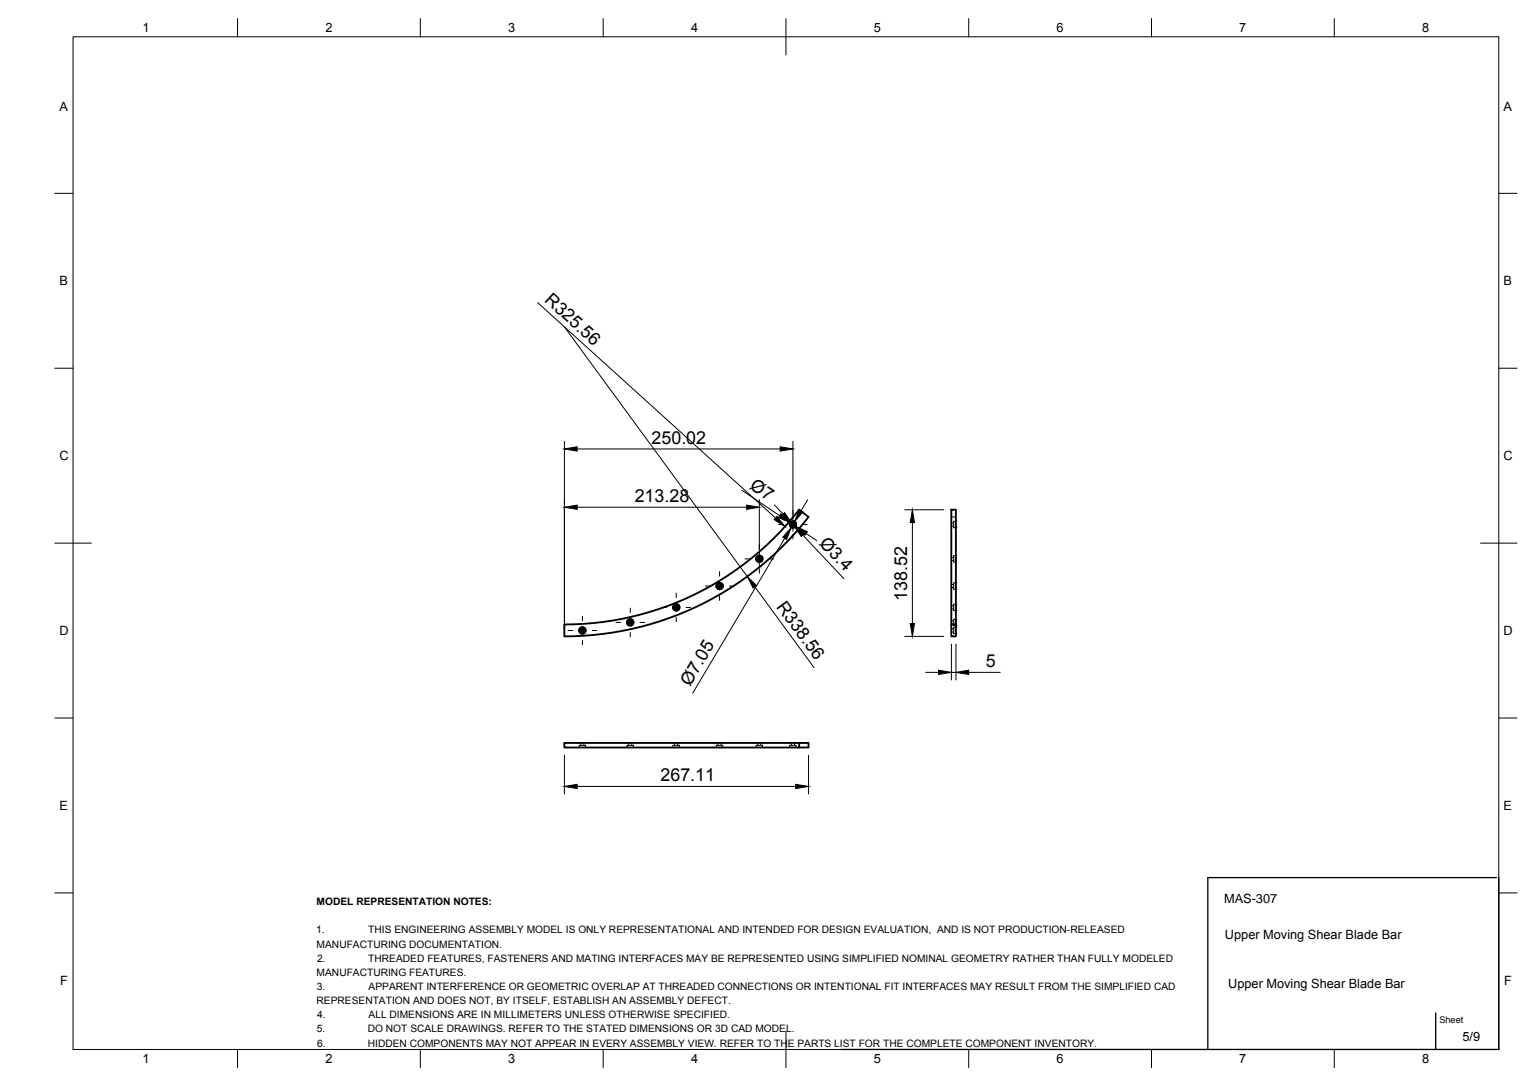
ISO-10303-21;
HEADER;
FILE_DESCRIPTION (('STEP AP214'),
    '1' );
FILE_NAME ('Upper Moving Shear Blade Bar.step',
    '2026-10-06T07:34:29',
    ( '' ),
    ( '' ),
    'SwSTEP 2.0',
    'SolidWorks 2025',
    '' );
FILE_SCHEMA (( 'AUTOMOTIVE_DESIGN' ));
ENDSEC;

DATA;
#5=CIRCLE ( 'NONE', #1538, 3.525000000000000355 ) ;
#15=CARTESIAN_POINT ( 'NONE',  ( 66.76535645333922275, 38.79159067395544014, 7.600000000000002309 ) ) ;
#20=DIRECTION ( 'NONE',  ( -0.000000000000000000, -0.000000000000000000, 1.000000000000000000 ) ) ;
#38=DIRECTION ( 'NONE',  ( 1.000000000000000000, 0.000000000000000000, 0.000000000000000000 ) ) ;
#47=CARTESIAN_POINT ( 'NONE',  ( 70.26535645333922275, 38.79159067395544014, 10.00000000000000178 ) ) ;
#51=DIRECTION ( 'NONE',  ( 1.000000000000000000, 0.000000000000000000, 0.000000000000000000 ) ) ;
#52=CARTESIAN_POINT ( 'NONE',  ( -36.49899788034579018, 48.72489408690345414, 5.000000000000000000 ) ) ;
#60=EDGE_CURVE ( 'NONE', #13786, #6568, #5831, .T. ) ;
#63=ORIENTED_EDGE ( 'NONE', *, *, #11844, .T. ) ;
#76=CARTESIAN_POINT ( 'NONE',  ( 70.26535645333922275, 38.79159067395544014, 7.600000000000002309 ) ) ;
#82=DIRECTION ( 'NONE',  ( -0.000000000000000000, -0.000000000000000000, 1.000000000000000000 ) ) ;
#84=DIRECTION ( 'NONE',  ( 1.000000000000000000, 0.000000000000000000, 0.000000000000000000 ) ) ;
#90=LINE ( 'NONE', #10937, #11841 ) ;
#97=CARTESIAN_POINT ( 'NONE',  ( -34.79899788034579444, 48.72489408690345414, 10.00000000000000178 ) ) ;
#109=DIRECTION ( 'NONE',  ( -0.000000000000000000, -0.000000000000000000, 1.000000000000000000 ) ) ;
#120=ADVANCED_FACE ( 'NONE', ( #7198 ), #13161, .F. ) ;
#143=ORIENTED_EDGE ( 'NONE', *, *, #13656, .T. ) ;
#158=VERTEX_POINT ( 'NONE', #7269 ) ;
#175=ORIENTED_EDGE ( 'NONE', *, *, #1719, .F. ) ;
#184=DIRECTION ( 'NONE',  ( -0.000000000000000000, -0.000000000000000000, 1.000000000000000000 ) ) ;
#191=AXIS2_PLACEMENT_3D ( 'NONE', #8581, #13373, #8730 ) ;
#197=DIRECTION ( 'NONE',  ( 1.000000000000000000, 0.000000000000000000, 0.000000000000000000 ) ) ;
#204=DIRECTION ( 'NONE',  ( 1.000000000000000000, 0.000000000000000000, 0.000000000000000000 ) ) ;
#218=EDGE_CURVE ( 'NONE', #11968, #7924, #4346, .T. ) ;
#256=VERTEX_POINT ( 'NONE', #7495 ) ;
#266=DIRECTION ( 'NONE',  ( -0.000000000000000000, -0.000000000000000000, 1.000000000000000000 ) ) ;
#269=MANIFOLD_SOLID_BREP ( 'Move Face1', #9158 ) ;
#270=LINE ( 'NONE', #1701, #14484 ) ;
#273=VECTOR ( 'NONE', #10509, 1000.000000000000000 ) ;
#287=FACE_OUTER_BOUND ( 'NONE', #14918, .T. ) ;
#302=DIRECTION ( 'NONE',  ( 1.000000000000000000, 0.000000000000000000, 0.000000000000000000 ) ) ;
#342=FACE_OUTER_BOUND ( 'NONE', #1259, .T. ) ;
#352=EDGE_LOOP ( 'NONE', ( #9480, #1820, #544, #3677 ) ) ;
#354=DIRECTION ( 'NONE',  ( -0.000000000000000000, -0.000000000000000000, 1.000000000000000000 ) ) ;
#372=FACE_OUTER_BOUND ( 'NONE', #12651, .T. ) ;
#376=CARTESIAN_POINT ( 'NONE',  ( 19.11029453487719110, 40.04259805664093363, 7.600000000000002309 ) ) ;
#388=FACE_BOUND ( 'NONE', #1673, .T. ) ;
#407=DIRECTION ( 'NONE',  ( -0.000000000000000000, -0.000000000000000000, 1.000000000000000000 ) ) ;
#412=DIRECTION ( 'NONE',  ( 1.000000000000000000, 0.000000000000000000, 0.000000000000000000 ) ) ;
#414=FACE_OUTER_BOUND ( 'NONE', #14323, .T. ) ;
#418=ADVANCED_FACE ( 'NONE', ( #10869 ), #4776, .F. ) ;
#430=FACE_OUTER_BOUND ( 'NONE', #4920, .T. ) ;
#439=ADVANCED_FACE ( 'NONE', ( #5527 ), #13887, .F. ) ;
#440=DIRECTION ( 'NONE',  ( 1.000000000000000000, 0.000000000000000000, 0.000000000000000000 ) ) ;
#447=ORIENTED_EDGE ( 'NONE', *, *, #8449, .T. ) ;
#452=CARTESIAN_POINT ( 'NONE',  ( 122.5806775638430253, 45.00321902537314145, 7.600000000000002309 ) ) ;
#453=AXIS2_PLACEMENT_3D ( 'NONE', #12309, #7594, #7753 ) ;
#454=VECTOR ( 'NONE', #11405, 1000.000000000000114 ) ;
#457=VERTEX_POINT ( 'NONE', #4861 ) ;
#475=DIRECTION ( 'NONE',  ( -1.000000000000000000, 0.000000000000000000, 0.000000000000000000 ) ) ;
#492=DIRECTION ( 'NONE',  ( 1.000000000000000000, 0.000000000000000000, 0.000000000000000000 ) ) ;
#493=CARTESIAN_POINT ( 'NONE',  ( -33.09899788034579160, 48.72489408690345414, 7.600000000000002309 ) ) ;
#507=LINE ( 'NONE', #14731, #10105 ) ;
#508=ORIENTED_EDGE ( 'NONE', *, *, #8880, .F. ) ;
#509=EDGE_LOOP ( 'NONE', ( #9428, #2544 ) ) ;
#511=CARTESIAN_POINT ( 'NONE',  ( 124.2806775638430281, 45.00321902537314145, 5.000000000000000000 ) ) ;
#538=CARTESIAN_POINT ( 'NONE',  ( 70.26535645333922275, 38.79159067395544014, 10.00000000000000178 ) ) ;
#540=FACE_OUTER_BOUND ( 'NONE', #6429, .T. ) ;
#544=ORIENTED_EDGE ( 'NONE', *, *, #8820, .T. ) ;
#551=ORIENTED_EDGE ( 'NONE', *, *, #13799, .F. ) ;
#556=SHAPE_REPRESENTATION ( 'Upper Moving Shear Blade Bar', ( #12337 ), #11555 ) ;
#569=DIRECTION ( 'NONE',  ( 1.000000000000000000, 0.000000000000000000, 0.000000000000000000 ) ) ;
#574=UNCERTAINTY_MEASURE_WITH_UNIT (LENGTH_MEASURE( 1.000000000000000082E-05 ), #14890, 'distance_accuracy_value', 'NONE');
#589=ORIENTED_EDGE ( 'NONE', *, *, #6377, .F. ) ;
#601=CIRCLE ( 'NONE', #13716, 3.500000000000003109 ) ;
#606=AXIS2_PLACEMENT_3D ( 'NONE', #2740, #184, #1548 ) ;
#622=EDGE_CURVE ( 'NONE', #2293, #7132, #13393, .T. ) ;
#633=CARTESIAN_POINT ( 'NONE',  ( -31.27399788034579586, 48.72489408690345414, 10.00000000000000178 ) ) ;
#656=CARTESIAN_POINT ( 'NONE',  ( -33.09899788034579871, 48.72489408690345414, 10.00000000000000178 ) ) ;
#675=DIRECTION ( 'NONE',  ( -0.000000000000000000, -0.000000000000000000, 1.000000000000000000 ) ) ;
#705=EDGE_CURVE ( 'NONE', #14207, #5229, #14437, .T. ) ;
#734=EDGE_CURVE ( 'NONE', #12823, #5329, #1812, .T. ) ;
#738=CARTESIAN_POINT ( 'NONE',  ( -105.7032403413611661, 68.63699971342407480, 10.00000000000000178 ) ) ;
#748=EDGE_LOOP ( 'NONE', ( #9743, #1718 ) ) ;
#749=ORIENTED_EDGE ( 'NONE', *, *, #705, .F. ) ;
#752=LINE ( 'NONE', #5511, #3482 ) ;
#753=CIRCLE ( 'NONE', #1005, 3.525000000000000355 ) ;
#754=AXIS2_PLACEMENT_3D ( 'NONE', #3682, #1381, #6219 ) ;
#762=AXIS2_PLACEMENT_3D ( 'NONE', #942, #1027, #8085 ) ;
#771=CARTESIAN_POINT ( 'NONE',  ( -85.27455057502459113, 65.19100426474074084, 10.00000000000000178 ) ) ;
#772=ORIENTED_EDGE ( 'NONE', *, *, #9707, .F. ) ;
#795=LINE ( 'NONE', #4513, #5561 ) ;
#803=DIRECTION ( 'NONE',  ( -0.000000000000000000, -0.000000000000000000, 1.000000000000000000 ) ) ;
#810=VERTEX_POINT ( 'NONE', #13328 ) ;
#828=VERTEX_POINT ( 'NONE', #6562 ) ;
#834=DIRECTION ( 'NONE',  ( -0.000000000000000000, 0.000000000000000000, 1.000000000000000000 ) ) ;
#837=VECTOR ( 'NONE', #9700, 1000.000000000000000 ) ;
#845=DIRECTION ( 'NONE',  ( 1.000000000000000000, 0.000000000000000000, 0.000000000000000000 ) ) ;
#847=AXIS2_PLACEMENT_3D ( 'NONE', #10566, #8058, #12846 ) ;
#872=CIRCLE ( 'NONE', #11474, 3.500000000000003109 ) ;
#875=DIRECTION ( 'NONE',  ( 1.000000000000000000, 0.000000000000000000, 0.000000000000000000 ) ) ;
#880=ORIENTED_EDGE ( 'NONE', *, *, #9050, .T. ) ;
#883=CARTESIAN_POINT ( 'NONE',  ( -31.27399788034579586, 48.72489408690345414, 10.00000000000000178 ) ) ;
#900=DIRECTION ( 'NONE',  ( -0.000000000000000000, -0.000000000000000000, -1.000000000000000000 ) ) ;
#911=ADVANCED_FACE ( 'NONE', ( #11682 ), #8886, .F. ) ;
#933=DIRECTION ( 'NONE',  ( -0.000000000000000000, -0.000000000000000000, 1.000000000000000000 ) ) ;
#935=VERTEX_POINT ( 'NONE', #2196 ) ;
#938=EDGE_CURVE ( 'NONE', #2958, #9645, #5088, .T. ) ;
#940=ORIENTED_EDGE ( 'NONE', *, *, #1886, .F. ) ;
#942=CARTESIAN_POINT ( 'NONE',  ( 172.5293059057019889, 61.25683321636181233, 7.600000000000002309 ) ) ;
#956=VERTEX_POINT ( 'NONE', #3310 ) ;
#976=EDGE_LOOP ( 'NONE', ( #1480, #10214, #12873, #13520 ) ) ;
#977=CARTESIAN_POINT ( 'NONE',  ( 71.96535645333923981, 38.79159067395544014, 7.600000000000002309 ) ) ;
#997=CARTESIAN_POINT ( 'NONE',  ( 176.0293059057019889, 61.25683321636181233, 7.600000000000002309 ) ) ;
#1005=AXIS2_PLACEMENT_3D ( 'NONE', #12927, #3078, #15361 ) ;
#1027=DIRECTION ( 'NONE',  ( -0.000000000000000000, -0.000000000000000000, 1.000000000000000000 ) ) ;
#1029=DIRECTION ( 'NONE',  ( 1.000000000000000000, 0.000000000000000000, 0.000000000000000000 ) ) ;
#1085=CARTESIAN_POINT ( 'NONE',  ( -34.79899788034579444, 48.72489408690345414, 7.600000000000002309 ) ) ;
#1096=EDGE_LOOP ( 'NONE', ( #7071, #14748 ) ) ;
#1098=VERTEX_POINT ( 'NONE', #10967 ) ;
#1117=ORIENTED_EDGE ( 'NONE', *, *, #218, .F. ) ;
#1118=LINE ( 'NONE', #14294, #8578 ) ;
#1125=EDGE_LOOP ( 'NONE', ( #7007, #5807 ) ) ;
#1139=FACE_OUTER_BOUND ( 'NONE', #12303, .T. ) ;
#1162=ORIENTED_EDGE ( 'NONE', *, *, #10778, .F. ) ;
#1167=FACE_BOUND ( 'NONE', #3663, .T. ) ;
#1168=CARTESIAN_POINT ( 'NONE',  ( 51.07686401294030532, 368.7106150007013525, 10.00000000000000178 ) ) ;
#1171=ORIENTED_EDGE ( 'NONE', *, *, #5302, .T. ) ;
#1179=CARTESIAN_POINT ( 'NONE',  ( -34.79899788034579444, 48.72489408690345414, 5.000000000000000000 ) ) ;
#1180=CARTESIAN_POINT ( 'NONE',  ( 119.0806775638430253, 45.00321902537314145, 10.00000000000000178 ) ) ;
#1185=DIRECTION ( 'NONE',  ( -0.000000000000000000, -0.000000000000000000, 1.000000000000000000 ) ) ;
#1189=CIRCLE ( 'NONE', #6262, 3.500000000000003109 ) ;
#1196=CIRCLE ( 'NONE', #10531, 1.700000000000007061 ) ;
#1204=ORIENTED_EDGE ( 'NONE', *, *, #5302, .F. ) ;
#1211=DIRECTION ( 'NONE',  ( -1.000000000000000000, 0.000000000000000000, 0.000000000000000000 ) ) ;
#1218=AXIS2_PLACEMENT_3D ( 'NONE', #1179, #3479, #13179 ) ;
#1222=ORIENTED_EDGE ( 'NONE', *, *, #4363, .T. ) ;
#1226=DIRECTION ( 'NONE',  ( -0.000000000000000000, -0.000000000000000000, 1.000000000000000000 ) ) ;
#1227=FACE_OUTER_BOUND ( 'NONE', #14901, .T. ) ;
#1256=CARTESIAN_POINT ( 'NONE',  ( 170.8293059057019718, 61.25683321636181233, 10.00000000000000178 ) ) ;
#1259=EDGE_LOOP ( 'NONE', ( #5459, #10454, #4600, #3411 ) ) ;
#1274=EDGE_LOOP ( 'NONE', ( #3424, #1499, #2007, #2831 ) ) ;
#1275=CARTESIAN_POINT ( 'NONE',  ( 17.41029453487719181, 40.04259805664093363, 7.600000000000002309 ) ) ;
#1286=CARTESIAN_POINT ( 'NONE',  ( 124.2806775638430281, 45.00321902537314145, 7.600000000000002309 ) ) ;
#1294=CARTESIAN_POINT ( 'NONE',  ( -81.74955057502458544, 65.19100426474074084, 10.00000000000000178 ) ) ;
#1305=DIRECTION ( 'NONE',  ( 1.000000000000000000, 0.000000000000000000, 0.000000000000000000 ) ) ;
#1325=FACE_BOUND ( 'NONE', #9221, .T. ) ;
#1341=CARTESIAN_POINT ( 'NONE',  ( 70.26535645333922275, 38.79159067395544014, 10.00000000000000178 ) ) ;
#1349=DIRECTION ( 'NONE',  ( -0.000000000000000000, -0.000000000000000000, -1.000000000000000000 ) ) ;
#1381=DIRECTION ( 'NONE',  ( -0.000000000000000000, -0.000000000000000000, 1.000000000000000000 ) ) ;
#1383=DIRECTION ( 'NONE',  ( 1.000000000000000000, 0.000000000000000000, 0.000000000000000000 ) ) ;
#1393=CARTESIAN_POINT ( 'NONE',  ( -31.29899788034579089, 48.72489408690345414, 7.600000000000002309 ) ) ;
#1396=CARTESIAN_POINT ( 'NONE',  ( 70.26535645333922275, 38.79159067395544014, 5.000000000000000000 ) ) ;
#1420=CARTESIAN_POINT ( 'NONE',  ( -34.79899788034579444, 48.72489408690345414, 10.00000000000000178 ) ) ;
#1426=VERTEX_POINT ( 'NONE', #8206 ) ;
#1446=DIRECTION ( 'NONE',  ( 1.000000000000000000, 0.000000000000000000, 0.000000000000000000 ) ) ;
#1463=ORIENTED_EDGE ( 'NONE', *, *, #6997, .F. ) ;
#1472=CARTESIAN_POINT ( 'NONE',  ( 122.5806775638430253, 45.00321902537314145, 10.00000000000000178 ) ) ;
#1476=CARTESIAN_POINT ( 'NONE',  ( -86.97455057502459397, 65.19100426474074084, 10.00000000000000178 ) ) ;
#1480=ORIENTED_EDGE ( 'NONE', *, *, #734, .F. ) ;
#1494=ORIENTED_EDGE ( 'NONE', *, *, #10730, .T. ) ;
#1499=ORIENTED_EDGE ( 'NONE', *, *, #9175, .T. ) ;
#1507=LINE ( 'NONE', #10999, #2120 ) ;
#1511=LINE ( 'NONE', #11231, #6713 ) ;
#1538=AXIS2_PLACEMENT_3D ( 'NONE', #14552, #13293, #7325 ) ;
#1548=DIRECTION ( 'NONE',  ( 1.000000000000000000, 0.000000000000000000, 0.000000000000000000 ) ) ;
#1553=ORIENTED_EDGE ( 'NONE', *, *, #12044, .T. ) ;
#1554=LINE ( 'NONE', #1787, #12369 ) ;
#1604=EDGE_CURVE ( 'NONE', #956, #13999, #11477, .T. ) ;
#1613=AXIS2_PLACEMENT_3D ( 'NONE', #12528, #5520, #1722 ) ;
#1620=ORIENTED_EDGE ( 'NONE', *, *, #11583, .F. ) ;
#1633=EDGE_CURVE ( 'NONE', #8949, #7872, #9856, .T. ) ;
#1634=AXIS2_PLACEMENT_3D ( 'NONE', #15188, #12908, #6927 ) ;
#1641=DIRECTION ( 'NONE',  ( -0.000000000000000000, 0.000000000000000000, 1.000000000000000000 ) ) ;
#1645=CYLINDRICAL_SURFACE ( 'NONE', #5383, 3.499999999999999556 ) ;
#1660=FACE_OUTER_BOUND ( 'NONE', #8338, .T. ) ;
#1673=EDGE_LOOP ( 'NONE', ( #11669, #7615 ) ) ;
#1682=EDGE_CURVE ( 'NONE', #5329, #12823, #13351, .T. ) ;
#1697=DIRECTION ( 'NONE',  ( -0.000000000000000000, -0.000000000000000000, 1.000000000000000000 ) ) ;
#1698=CIRCLE ( 'NONE', #3471, 3.499999999999999556 ) ;
#1701=CARTESIAN_POINT ( 'NONE',  ( -31.29899788034579089, 48.72489408690345414, 10.00000000000000178 ) ) ;
#1706=PRODUCT_DEFINITION_SHAPE ( 'NONE', 'NONE',  #4976 ) ;
#1713=AXIS2_PLACEMENT_3D ( 'NONE', #5111, #12137, #8746 ) ;
#1718=ORIENTED_EDGE ( 'NONE', *, *, #4489, .F. ) ;
#1719=EDGE_CURVE ( 'NONE', #3938, #7406, #5234, .T. ) ;
#1722=DIRECTION ( 'NONE',  ( 1.000000000000000000, 0.000000000000000000, 0.000000000000000000 ) ) ;
#1726=EDGE_LOOP ( 'NONE', ( #15460, #12803, #6817, #4219 ) ) ;
#1741=VECTOR ( 'NONE', #7234, 1000.000000000000000 ) ;
#1759=DIRECTION ( 'NONE',  ( 1.000000000000000000, 0.000000000000000000, 0.000000000000000000 ) ) ;
#1781=CARTESIAN_POINT ( 'NONE',  ( 172.5293059057019889, 61.25683321636181233, 10.00000000000000178 ) ) ;
#1783=CARTESIAN_POINT ( 'NONE',  ( 13.91029453487719181, 40.04259805664093363, 7.600000000000002309 ) ) ;
#1787=CARTESIAN_POINT ( 'NONE',  ( 66.76535645333922275, 38.79159067395544014, 10.00000000000000178 ) ) ;
#1812=CIRCLE ( 'NONE', #6623, 3.499999999999996003 ) ;
#1816=AXIS2_PLACEMENT_3D ( 'NONE', #3969, #8888, #13595 ) ;
#1820=ORIENTED_EDGE ( 'NONE', *, *, #9243, .T. ) ;
#1822=MECHANICAL_DESIGN_GEOMETRIC_PRESENTATION_REPRESENTATION('',(#4599),#12887);
#1834=DIRECTION ( 'NONE',  ( 0.000000000000000000, 0.000000000000000000, -1.000000000000000000 ) ) ;
#1842=ORIENTED_EDGE ( 'NONE', *, *, #14993, .F. ) ;
#1859=EDGE_LOOP ( 'NONE', ( #2042, #2199, #11914, #1842 ) ) ;
#1861=EDGE_CURVE ( 'NONE', #12197, #8972, #3037, .T. ) ;
#1862=ORIENTED_EDGE ( 'NONE', *, *, #6839, .F. ) ;
#1873=CARTESIAN_POINT ( 'NONE',  ( 174.2293059057019775, 61.25683321636181233, 5.000000000000000000 ) ) ;
#1886=EDGE_CURVE ( 'NONE', #8972, #935, #795, .T. ) ;
#1903=CARTESIAN_POINT ( 'NONE',  ( 172.5293059057019889, 61.25683321636181233, 7.600000000000002309 ) ) ;
#1937=ORIENTED_EDGE ( 'NONE', *, *, #4142, .F. ) ;
#1947=EDGE_CURVE ( 'NONE', #11858, #256, #2789, .T. ) ;
#1974=AXIS2_PLACEMENT_3D ( 'NONE', #14287, #2218, #11936 ) ;
#1978=LINE ( 'NONE', #633, #12056 ) ;
#1981=ORIENTED_EDGE ( 'NONE', *, *, #8820, .F. ) ;
#1987=ADVANCED_FACE ( 'NONE', ( #6101 ), #7291, .F. ) ;
#2001=EDGE_LOOP ( 'NONE', ( #3858, #3321, #12575, #4549 ) ) ;
#2002=AXIS2_PLACEMENT_3D ( 'NONE', #2956, #8720, #7775 ) ;
#2007=ORIENTED_EDGE ( 'NONE', *, *, #2102, .T. ) ;
#2039=EDGE_CURVE ( 'NONE', #7454, #8789, #10609, .T. ) ;
#2042=ORIENTED_EDGE ( 'NONE', *, *, #1947, .F. ) ;
#2059=AXIS2_PLACEMENT_3D ( 'NONE', #15441, #9540, #845 ) ;
#2074=ORIENTED_EDGE ( 'NONE', *, *, #6696, .F. ) ;
#2085=AXIS2_PLACEMENT_3D ( 'NONE', #10680, #1185, #12089 ) ;
#2096=DIRECTION ( 'NONE',  ( 1.000000000000000000, 0.000000000000000000, 0.000000000000000000 ) ) ;
#2102=EDGE_CURVE ( 'NONE', #3731, #7373, #13620, .T. ) ;
#2120=VECTOR ( 'NONE', #1349, 1000.000000000000000 ) ;
#2126=CARTESIAN_POINT ( 'NONE',  ( 70.26535645333922275, 38.79159067395544014, 7.600000000000002309 ) ) ;
#2141=CIRCLE ( 'NONE', #3913, 1.700000000000000178 ) ;
#2148=ADVANCED_FACE ( 'NONE', ( #12468 ), #14629, .F. ) ;
#2150=VERTEX_POINT ( 'NONE', #376 ) ;
#2172=PLANE ( 'NONE',  #4664 ) ;
#2175=LINE ( 'NONE', #4545, #12545 ) ;
#2181=ORIENTED_EDGE ( 'NONE', *, *, #60, .F. ) ;
#2184=CARTESIAN_POINT ( 'NONE',  ( 0.000000000000000000, 0.000000000000000000, 10.00000000000000178 ) ) ;
#2189=EDGE_CURVE ( 'NONE', #12185, #15218, #2286, .T. ) ;
#2195=CARTESIAN_POINT ( 'NONE',  ( 124.2806775638430281, 45.00321902537314145, 10.00000000000000178 ) ) ;
#2196=CARTESIAN_POINT ( 'NONE',  ( -81.77455057502459113, 65.19100426474074084, 9.975000000000001421 ) ) ;
#2199=ORIENTED_EDGE ( 'NONE', *, *, #12619, .T. ) ;
#2201=CIRCLE ( 'NONE', #13024, 1.700000000000007061 ) ;
#2218=DIRECTION ( 'NONE',  ( -0.000000000000000000, -0.000000000000000000, 1.000000000000000000 ) ) ;
#2237=ORIENTED_EDGE ( 'NONE', *, *, #11806, .T. ) ;
#2249=EDGE_LOOP ( 'NONE', ( #9218, #10170, #8571, #13907 ) ) ;
#2257=AXIS2_PLACEMENT_3D ( 'NONE', #12770, #9315, #9238 ) ;
#2279=CARTESIAN_POINT ( 'NONE',  ( 186.1005832062958234, 72.46888774096882457, 10.00000000000000178 ) ) ;
#2286=CIRCLE ( 'NONE', #9349, 3.500000000000003109 ) ;
#2293=VERTEX_POINT ( 'NONE', #3231 ) ;
#2307=VECTOR ( 'NONE', #6012, 1000.000000000000000 ) ;
#2311=FACE_BOUND ( 'NONE', #3877, .T. ) ;
#2335=CARTESIAN_POINT ( 'NONE',  ( 13.91029453487719181, 40.04259805664093363, 9.975000000000001421 ) ) ;
#2342=EDGE_LOOP ( 'NONE', ( #3842, #7278 ) ) ;
#2387=EDGE_CURVE ( 'NONE', #7406, #810, #9610, .T. ) ;
#2391=VECTOR ( 'NONE', #14651, 1000.000000000000000 ) ;
#2432=ORIENTED_EDGE ( 'NONE', *, *, #13357, .T. ) ;
#2433=EDGE_CURVE ( 'NONE', #10355, #6706, #5971, .T. ) ;
#2437=CYLINDRICAL_SURFACE ( 'NONE', #10901, 3.500000000000003109 ) ;
#2451=ORIENTED_EDGE ( 'NONE', *, *, #7116, .T. ) ;
#2487=FACE_BOUND ( 'NONE', #4495, .T. ) ;
#2495=CIRCLE ( 'NONE', #3505, 3.500000000000003109 ) ;
#2497=DIRECTION ( 'NONE',  ( -0.000000000000000000, -0.000000000000000000, 1.000000000000000000 ) ) ;
#2506=CARTESIAN_POINT ( 'NONE',  ( 13.91029453487719181, 40.04259805664093363, 10.00000000000000178 ) ) ;
#2512=ADVANCED_FACE ( 'NONE', ( #13319, #1167, #1325, #5997, #3781, #4967, #10818 ), #15607, .F. ) ;
#2519=CIRCLE ( 'NONE', #9844, 1.700000000000000178 ) ;
#2524=ORIENTED_EDGE ( 'NONE', *, *, #1604, .F. ) ;
#2544=ORIENTED_EDGE ( 'NONE', *, *, #3841, .T. ) ;
#2558=CARTESIAN_POINT ( 'NONE',  ( -36.49899788034579728, 48.72489408690345414, 7.600000000000002309 ) ) ;
#2561=DIRECTION ( 'NONE',  ( -0.000000000000000000, -0.000000000000000000, 1.000000000000000000 ) ) ;
#2562=CARTESIAN_POINT ( 'NONE',  ( 17.41029453487719181, 40.04259805664093363, 10.00000000000000178 ) ) ;
#2619=DIRECTION ( 'NONE',  ( -0.000000000000000000, -0.000000000000000000, 1.000000000000000000 ) ) ;
#2658=DIRECTION ( 'NONE',  ( 1.000000000000000000, 0.000000000000000000, 0.000000000000000000 ) ) ;
#2659=DIRECTION ( 'NONE',  ( 1.000000000000000000, 0.000000000000000000, 0.000000000000000000 ) ) ;
#2664=EDGE_CURVE ( 'NONE', #6169, #1426, #14784, .T. ) ;
#2671=AXIS2_PLACEMENT_3D ( 'NONE', #13362, #2561, #2715 ) ;
#2674=CARTESIAN_POINT ( 'NONE',  ( 172.5293059057019889, 61.25683321636181233, 9.975000000000001421 ) ) ;
#2694=EDGE_CURVE ( 'NONE', #3938, #8914, #2201, .T. ) ;
#2704=CARTESIAN_POINT ( 'NONE',  ( 126.1056775638430310, 45.00321902537314145, 10.00000000000000178 ) ) ;
#2708=CARTESIAN_POINT ( 'NONE',  ( 119.0806775638430253, 45.00321902537314145, 7.600000000000002309 ) ) ;
#2711=DIRECTION ( 'NONE',  ( 1.000000000000000000, 0.000000000000000000, 0.000000000000000000 ) ) ;
#2715=DIRECTION ( 'NONE',  ( 1.000000000000000000, 0.000000000000000000, 0.000000000000000000 ) ) ;
#2724=AXIS2_PLACEMENT_3D ( 'NONE', #7525, #11464, #5149 ) ;
#2737=DIRECTION ( 'NONE',  ( 1.000000000000000000, 0.000000000000000000, 0.000000000000000000 ) ) ;
#2740=CARTESIAN_POINT ( 'NONE',  ( 172.5293059057019889, 61.25683321636181233, 10.00000000000000178 ) ) ;
#2776=DIRECTION ( 'NONE',  ( -0.000000000000000000, -0.000000000000000000, 1.000000000000000000 ) ) ;
#2789=CIRCLE ( 'NONE', #13612, 3.499999999999999556 ) ;
#2797=DIRECTION ( 'NONE',  ( -0.000000000000000000, -0.000000000000000000, 1.000000000000000000 ) ) ;
#2831=ORIENTED_EDGE ( 'NONE', *, *, #14143, .F. ) ;
#2832=ORIENTED_EDGE ( 'NONE', *, *, #14560, .F. ) ;
#2841=ORIENTED_EDGE ( 'NONE', *, *, #14264, .F. ) ;
#2843=PRODUCT_DEFINITION_CONTEXT ( 'detailed design', #12900, 'design' ) ;
#2854=DIRECTION ( 'NONE',  ( -0.000000000000000000, -0.000000000000000000, 1.000000000000000000 ) ) ;
#2857=DIRECTION ( 'NONE',  ( -0.000000000000000000, -0.000000000000000000, 1.000000000000000000 ) ) ;
#2859=EDGE_CURVE ( 'NONE', #8410, #11968, #3608, .T. ) ;
#2863=CARTESIAN_POINT ( 'NONE',  ( 20.91029453487719181, 40.04259805664093363, 10.00000000000000178 ) ) ;
#2881=AXIS2_PLACEMENT_3D ( 'NONE', #13610, #12578, #412 ) ;
#2890=ORIENTED_EDGE ( 'NONE', *, *, #10778, .T. ) ;
#2895=ADVANCED_FACE ( 'NONE', ( #1227 ), #5821, .F. ) ;
#2913=DIRECTION ( 'NONE',  ( -0.7071067811864983899, 8.659560562354331352E-17, 0.7071067811865966446 ) ) ;
#2940=ORIENTED_EDGE ( 'NONE', *, *, #11588, .F. ) ;
#2948=DIRECTION ( 'NONE',  ( 1.000000000000000000, 0.000000000000000000, 0.000000000000000000 ) ) ;
#2950=ADVANCED_FACE ( 'NONE', ( #14790 ), #4437, .F. ) ;
#2956=CARTESIAN_POINT ( 'NONE',  ( -34.79899788034579444, 48.72489408690345414, 10.00000000000000178 ) ) ;
#2958=VERTEX_POINT ( 'NONE', #493 ) ;
#2972=CIRCLE ( 'NONE', #10288, 1.700000000000000178 ) ;
#2974=ORIENTED_EDGE ( 'NONE', *, *, #14811, .F. ) ;
#2975=CYLINDRICAL_SURFACE ( 'NONE', #10213, 1.700000000000007061 ) ;
#3005=CARTESIAN_POINT ( 'NONE',  ( 170.8293059057019718, 61.25683321636181233, 7.600000000000002309 ) ) ;
#3021=ORIENTED_EDGE ( 'NONE', *, *, #4796, .T. ) ;
#3023=FACE_OUTER_BOUND ( 'NONE', #9962, .T. ) ;
#3031=DIRECTION ( 'NONE',  ( -0.000000000000000000, 0.000000000000000000, 1.000000000000000000 ) ) ;
#3037=CIRCLE ( 'NONE', #5050, 3.500000000000003109 ) ;
#3047=DIRECTION ( 'NONE',  ( 0.000000000000000000, 0.000000000000000000, -1.000000000000000000 ) ) ;
#3063=CARTESIAN_POINT ( 'NONE',  ( -33.09899788034579160, 48.72489408690345414, 7.600000000000002309 ) ) ;
#3078=DIRECTION ( 'NONE',  ( -0.000000000000000000, -0.000000000000000000, 1.000000000000000000 ) ) ;
#3106=EDGE_CURVE ( 'NONE', #6568, #2293, #8667, .T. ) ;
#3140=DIRECTION ( 'NONE',  ( 1.000000000000000000, 0.000000000000000000, 0.000000000000000000 ) ) ;
#3154=EDGE_CURVE ( 'NONE', #15074, #14924, #8737, .T. ) ;
#3162=ORIENTED_EDGE ( 'NONE', *, *, #11620, .F. ) ;
#3173=DIRECTION ( 'NONE',  ( -0.7071067811864983899, 8.659560562354331352E-17, 0.7071067811865966446 ) ) ;
#3212=FACE_BOUND ( 'NONE', #10839, .T. ) ;
#3219=CARTESIAN_POINT ( 'NONE',  ( 122.5806775638430253, 45.00321902537314145, 5.000000000000000000 ) ) ;
#3224=ORIENTED_EDGE ( 'NONE', *, *, #938, .T. ) ;
#3231=CARTESIAN_POINT ( 'NONE',  ( 169.0293059057019889, 61.25683321636181233, 9.975000000000001421 ) ) ;
#3248=DIRECTION ( 'NONE',  ( 1.000000000000000000, 0.000000000000000000, 0.000000000000000000 ) ) ;
#3251=AXIS2_PLACEMENT_3D ( 'NONE', #7788, #407, #5244 ) ;
#3256=CARTESIAN_POINT ( 'NONE',  ( 176.0543059057019661, 61.25683321636181233, 10.00000000000000178 ) ) ;
#3257=DIRECTION ( 'NONE',  ( 1.000000000000000000, 0.000000000000000000, 0.000000000000000000 ) ) ;
#3280=VECTOR ( 'NONE', #2497, 1000.000000000000000 ) ;
#3281=ORIENTED_EDGE ( 'NONE', *, *, #2039, .F. ) ;
#3295=AXIS2_PLACEMENT_3D ( 'NONE', #76, #10841, #12238 ) ;
#3310=CARTESIAN_POINT ( 'NONE',  ( 126.0806775638430253, 45.00321902537314145, 9.975000000000001421 ) ) ;
#3315=DIRECTION ( 'NONE',  ( -0.000000000000000000, -0.000000000000000000, 1.000000000000000000 ) ) ;
#3321=ORIENTED_EDGE ( 'NONE', *, *, #705, .T. ) ;
#3330=ORIENTED_EDGE ( 'NONE', *, *, #6997, .T. ) ;
#3331=DIRECTION ( 'NONE',  ( 0.7071067811865965336, 0.000000000000000000, 0.7071067811864985009 ) ) ;
#3372=DIRECTION ( 'NONE',  ( -0.000000000000000000, -0.000000000000000000, 1.000000000000000000 ) ) ;
#3381=DIRECTION ( 'NONE',  ( -0.000000000000000000, -0.000000000000000000, 1.000000000000000000 ) ) ;
#3405=DIRECTION ( 'NONE',  ( -0.000000000000000000, -0.000000000000000000, 1.000000000000000000 ) ) ;
#3411=ORIENTED_EDGE ( 'NONE', *, *, #3721, .F. ) ;
#3424=ORIENTED_EDGE ( 'NONE', *, *, #7515, .F. ) ;
#3426=UNCERTAINTY_MEASURE_WITH_UNIT (LENGTH_MEASURE( 1.000000000000000082E-05 ), #15053, 'distance_accuracy_value', 'NONE');
#3448=EDGE_LOOP ( 'NONE', ( #10788, #8936, #4929, #9659 ) ) ;
#3469=EDGE_CURVE ( 'NONE', #1098, #8246, #10995, .T. ) ;
#3471=AXIS2_PLACEMENT_3D ( 'NONE', #10125, #14919, #12058 ) ;
#3479=DIRECTION ( 'NONE',  ( -0.000000000000000000, 0.000000000000000000, 1.000000000000000000 ) ) ;
#3482=VECTOR ( 'NONE', #12835, 1000.000000000000000 ) ;
#3494=CARTESIAN_POINT ( 'NONE',  ( -88.77455057502459113, 65.19100426474074084, 7.600000000000002309 ) ) ;
#3496=DIRECTION ( 'NONE',  ( -0.000000000000000000, -0.000000000000000000, 1.000000000000000000 ) ) ;
#3505=AXIS2_PLACEMENT_3D ( 'NONE', #10343, #13968, #11607 ) ;
#3541=ORIENTED_EDGE ( 'NONE', *, *, #11754, .F. ) ;
#3548=LINE ( 'NONE', #3256, #9749 ) ;
#3550=ADVANCED_FACE ( 'NONE', ( #10290, #5631 ), #7700, .F. ) ;
#3584=ADVANCED_BREP_SHAPE_REPRESENTATION ( '', ( #269, #12337 ), #11555 ) ;
#3608=LINE ( 'NONE', #4631, #9248 ) ;
#3621=FACE_OUTER_BOUND ( 'NONE', #13646, .T. ) ;
#3641=ORIENTED_EDGE ( 'NONE', *, *, #11588, .T. ) ;
#3645=ADVANCED_FACE ( 'NONE', ( #4195 ), #11508, .F. ) ;
#3647=DIRECTION ( 'NONE',  ( 0.4147405137080060755, -0.9099397267342597129, 0.000000000000000000 ) ) ;
#3663=EDGE_LOOP ( 'NONE', ( #11878, #8174 ) ) ;
#3677=ORIENTED_EDGE ( 'NONE', *, *, #11806, .F. ) ;
#3682=CARTESIAN_POINT ( 'NONE',  ( 122.5806775638430253, 45.00321902537314145, 10.00000000000000178 ) ) ;
#3706=ORIENTED_EDGE ( 'NONE', *, *, #4142, .T. ) ;
#3715=DIRECTION ( 'NONE',  ( 1.000000000000000000, 0.000000000000000000, 0.000000000000000000 ) ) ;
#3721=EDGE_CURVE ( 'NONE', #7132, #8246, #3548, .T. ) ;
#3723=ORIENTED_EDGE ( 'NONE', *, *, #9522, .F. ) ;
#3731=VERTEX_POINT ( 'NONE', #13244 ) ;
#3732=EDGE_LOOP ( 'NONE', ( #12108, #1204 ) ) ;
#3749=CARTESIAN_POINT ( 'NONE',  ( 66.74035645333923128, 38.79159067395544014, 10.00000000000000178 ) ) ;
#3752=CARTESIAN_POINT ( 'NONE',  ( -85.27455057502459113, 65.19100426474074084, 5.000000000000000000 ) ) ;
#3778=DIRECTION ( 'NONE',  ( -0.000000000000000000, -0.000000000000000000, 1.000000000000000000 ) ) ;
#3781=FACE_BOUND ( 'NONE', #6342, .T. ) ;
#3801=DIRECTION ( 'NONE',  ( -0.000000000000000000, -0.000000000000000000, 1.000000000000000000 ) ) ;
#3804=ADVANCED_FACE ( 'NONE', ( #3023 ), #10211, .F. ) ;
#3809=ORIENTED_EDGE ( 'NONE', *, *, #9522, .T. ) ;
#3821=ORIENTED_EDGE ( 'NONE', *, *, #14885, .F. ) ;
#3841=EDGE_CURVE ( 'NONE', #14207, #13704, #11817, .T. ) ;
#3842=ORIENTED_EDGE ( 'NONE', *, *, #11844, .F. ) ;
#3850=AXIS2_PLACEMENT_3D ( 'NONE', #11150, #2857, #302 ) ;
#3856=ORIENTED_EDGE ( 'NONE', *, *, #11167, .F. ) ;
#3858=ORIENTED_EDGE ( 'NONE', *, *, #3841, .F. ) ;
#3859=DIRECTION ( 'NONE',  ( 1.000000000000000000, 0.000000000000000000, 0.000000000000000000 ) ) ;
#3863=CARTESIAN_POINT ( 'NONE',  ( -88.77455057502459113, 65.19100426474074084, 10.00000000000000178 ) ) ;
#3877=EDGE_LOOP ( 'NONE', ( #1117, #14798 ) ) ;
#3900=FACE_OUTER_BOUND ( 'NONE', #3960, .T. ) ;
#3913=AXIS2_PLACEMENT_3D ( 'NONE', #12727, #11403, #569 ) ;
#3914=DIRECTION ( 'NONE',  ( -1.000000000000000000, 0.000000000000000000, -0.000000000000000000 ) ) ;
#3919=EDGE_CURVE ( 'NONE', #6568, #13786, #11566, .T. ) ;
#3937=AXIS2_PLACEMENT_3D ( 'NONE', #7862, #1834, #11547 ) ;
#3938=VERTEX_POINT ( 'NONE', #6741 ) ;
#3960=EDGE_LOOP ( 'NONE', ( #15052, #9761, #3641, #10584 ) ) ;
#3962=DIRECTION ( 'NONE',  ( -0.000000000000000000, 0.000000000000000000, 1.000000000000000000 ) ) ;
#3969=CARTESIAN_POINT ( 'NONE',  ( 51.07686401294030532, 368.7106150007013525, 10.00000000000000178 ) ) ;
#3979=VERTEX_POINT ( 'NONE', #10281 ) ;
#3981=EDGE_CURVE ( 'NONE', #2293, #1098, #10515, .T. ) ;
#3995=DIRECTION ( 'NONE',  ( -0.000000000000000000, -0.000000000000000000, 1.000000000000000000 ) ) ;
#4004=EDGE_CURVE ( 'NONE', #8914, #810, #8244, .T. ) ;
#4007=AXIS2_PLACEMENT_3D ( 'NONE', #7699, #5082, #475 ) ;
#4013=CARTESIAN_POINT ( 'NONE',  ( -34.79899788034579444, 48.72489408690345414, 9.975000000000001421 ) ) ;
#4021=EDGE_CURVE ( 'NONE', #5329, #8949, #1978, .T. ) ;
#4022=EDGE_LOOP ( 'NONE', ( #6936, #12113, #4860, #6629 ) ) ;
#4031=ORIENTED_EDGE ( 'NONE', *, *, #8964, .F. ) ;
#4032=LINE ( 'NONE', #2863, #9200 ) ;
#4042=CIRCLE ( 'NONE', #762, 1.700000000000007061 ) ;
#4045=DIRECTION ( 'NONE',  ( 0.7071067811864983899, 0.000000000000000000, 0.7071067811865966446 ) ) ;
#4046=FACE_OUTER_BOUND ( 'NONE', #9753, .T. ) ;
#4072=CYLINDRICAL_SURFACE ( 'NONE', #606, 3.500000000000003109 ) ;
#4090=COLOUR_RGB ( '', 0.66274510, 0.83137255, 0.94901961) ;
#4099=CYLINDRICAL_SURFACE ( 'NONE', #453, 1.699999999999993072 ) ;
#4103=DIRECTION ( 'NONE',  ( -0.000000000000000000, -0.000000000000000000, 1.000000000000000000 ) ) ;
#4105=AXIS2_PLACEMENT_3D ( 'NONE', #6100, #13257, #3715 ) ;
#4110=ADVANCED_FACE ( 'NONE', ( #5859 ), #10752, .F. ) ;
#4142=EDGE_CURVE ( 'NONE', #6706, #10355, #12813, .T. ) ;
#4144=ORIENTED_EDGE ( 'NONE', *, *, #5726, .F. ) ;
#4149=ORIENTED_EDGE ( 'NONE', *, *, #14811, .T. ) ;
#4167=ORIENTED_EDGE ( 'NONE', *, *, #12126, .T. ) ;
#4177=DIRECTION ( 'NONE',  ( -0.000000000000000000, -0.000000000000000000, 1.000000000000000000 ) ) ;
#4183=ORIENTED_EDGE ( 'NONE', *, *, #9927, .T. ) ;
#4195=FACE_OUTER_BOUND ( 'NONE', #4022, .T. ) ;
#4203=ORIENTED_EDGE ( 'NONE', *, *, #8449, .F. ) ;
#4215=DIRECTION ( 'NONE',  ( -0.000000000000000000, -0.000000000000000000, 1.000000000000000000 ) ) ;
#4216=VECTOR ( 'NONE', #15519, 1000.000000000000000 ) ;
#4219=ORIENTED_EDGE ( 'NONE', *, *, #14560, .T. ) ;
#4237=AXIS2_PLACEMENT_3D ( 'NONE', #11236, #8875, #2948 ) ;
#4267=ADVANCED_FACE ( 'NONE', ( #11142 ), #4099, .F. ) ;
#4274=DIRECTION ( 'NONE',  ( 1.000000000000000000, 0.000000000000000000, 0.000000000000000000 ) ) ;
#4276=LINE ( 'NONE', #4514, #6057 ) ;
#4285=VECTOR ( 'NONE', #6532, 1000.000000000000000 ) ;
#4327=( NAMED_UNIT ( * ) SI_UNIT ( $, .STERADIAN. ) SOLID_ANGLE_UNIT ( ) );
#4346=CIRCLE ( 'NONE', #12913, 1.700000000000007061 ) ;
#4350=VERTEX_POINT ( 'NONE', #12932 ) ;
#4363=EDGE_CURVE ( 'NONE', #457, #14684, #2495, .T. ) ;
#4379=CIRCLE ( 'NONE', #1613, 1.700000000000007061 ) ;
#4394=CARTESIAN_POINT ( 'NONE',  ( -38.32399788034579302, 48.72489408690345414, 10.00000000000000178 ) ) ;
#4421=CARTESIAN_POINT ( 'NONE',  ( 13.88529453487718968, 40.04259805664093363, 10.00000000000000178 ) ) ;
#4433=CARTESIAN_POINT ( 'NONE',  ( 17.41029453487719181, 40.04259805664093363, 7.600000000000002309 ) ) ;
#4437=CONICAL_SURFACE ( 'NONE', #13255, 3.525000000000000355, 0.7853981633973787790 ) ;
#4449=CARTESIAN_POINT ( 'NONE',  ( 19.11029453487719110, 40.04259805664093363, 5.000000000000000000 ) ) ;
#4457=FACE_OUTER_BOUND ( 'NONE', #976, .T. ) ;
#4465=VERTEX_POINT ( 'NONE', #2279 ) ;
#4485=LINE ( 'NONE', #4571, #15396 ) ;
#4489=EDGE_CURVE ( 'NONE', #7872, #8949, #13030, .T. ) ;
#4495=EDGE_LOOP ( 'NONE', ( #12349, #3821 ) ) ;
#4507=CARTESIAN_POINT ( 'NONE',  ( 68.56535645333921991, 38.79159067395544014, 10.00000000000000178 ) ) ;
#4513=CARTESIAN_POINT ( 'NONE',  ( -81.77455057502459113, 65.19100426474074084, 10.00000000000000178 ) ) ;
#4514=CARTESIAN_POINT ( 'NONE',  ( 176.0293059057019889, 61.25683321636181233, 10.00000000000000178 ) ) ;
#4529=AXIS2_PLACEMENT_3D ( 'NONE', #5125, #7581, #14665 ) ;
#4542=EDGE_LOOP ( 'NONE', ( #3723, #13412 ) ) ;
#4543=FACE_OUTER_BOUND ( 'NONE', #2001, .T. ) ;
#4545=CARTESIAN_POINT ( 'NONE',  ( -111.2071507613730290, 58.10263819636593041, 5.000000000000000000 ) ) ;
#4549=ORIENTED_EDGE ( 'NONE', *, *, #12126, .F. ) ;
#4553=VECTOR ( 'NONE', #6468, 1000.000000000000000 ) ;
#4554=DIRECTION ( 'NONE',  ( 1.000000000000000000, 0.000000000000000000, 0.000000000000000000 ) ) ;
#4561=AXIS2_PLACEMENT_3D ( 'NONE', #7855, #10444, #11391 ) ;
#4564=CARTESIAN_POINT ( 'NONE',  ( 170.8293059057019718, 61.25683321636181233, 5.000000000000000000 ) ) ;
#4568=CARTESIAN_POINT ( 'NONE',  ( 0.000000000000000000, 0.000000000000000000, 0.000000000000000000 ) ) ;
#4571=CARTESIAN_POINT ( 'NONE',  ( 181.4384305232223369, 82.69763993231136112, 10.00000000000000178 ) ) ;
#4599=STYLED_ITEM ( 'NONE', ( #12451 ), #269 ) ;
#4600=ORIENTED_EDGE ( 'NONE', *, *, #3469, .T. ) ;
#4630=FACE_BOUND ( 'NONE', #15114, .T. ) ;
#4631=CARTESIAN_POINT ( 'NONE',  ( -83.57455057502457407, 65.19100426474074084, 10.00000000000000178 ) ) ;
#4646=CARTESIAN_POINT ( 'NONE',  ( 172.5293059057019889, 61.25683321636181233, 7.600000000000002309 ) ) ;
#4649=EDGE_CURVE ( 'NONE', #7132, #2293, #1189, .T. ) ;
#4651=VECTOR ( 'NONE', #900, 1000.000000000000000 ) ;
#4664=AXIS2_PLACEMENT_3D ( 'NONE', #977, #15498, #10628 ) ;
#4675=DIRECTION ( 'NONE',  ( 1.000000000000000000, 0.000000000000000000, 0.000000000000000000 ) ) ;
#4705=ORIENTED_EDGE ( 'NONE', *, *, #3919, .T. ) ;
#4708=DIRECTION ( 'NONE',  ( 1.000000000000000000, 0.000000000000000000, 0.000000000000000000 ) ) ;
#4711=ADVANCED_FACE ( 'NONE', ( #430 ), #13299, .F. ) ;
#4725=DIRECTION ( 'NONE',  ( 1.000000000000000000, 0.000000000000000000, 0.000000000000000000 ) ) ;
#4750=AXIS2_PLACEMENT_3D ( 'NONE', #1903, #6973, #3248 ) ;
#4752=CARTESIAN_POINT ( 'NONE',  ( -83.57455057502457407, 65.19100426474074084, 7.600000000000002309 ) ) ;
#4758=CARTESIAN_POINT ( 'NONE',  ( -85.27455057502459113, 65.19100426474074084, 7.600000000000002309 ) ) ;
#4776=CYLINDRICAL_SURFACE ( 'NONE', #14654, 1.699999999999993072 ) ;
#4777=DIRECTION ( 'NONE',  ( -0.000000000000000000, -0.000000000000000000, 1.000000000000000000 ) ) ;
#4792=CIRCLE ( 'NONE', #6821, 3.525000000000000355 ) ;
#4793=CONICAL_SURFACE ( 'NONE', #4529, 3.525000000000000355, 0.7853981633973787790 ) ;
#4796=EDGE_CURVE ( 'NONE', #7924, #11968, #10295, .T. ) ;
#4810=DIRECTION ( 'NONE',  ( 1.000000000000000000, 0.000000000000000000, 0.000000000000000000 ) ) ;
#4847=ORIENTED_EDGE ( 'NONE', *, *, #11767, .T. ) ;
#4860=ORIENTED_EDGE ( 'NONE', *, *, #14993, .T. ) ;
#4861=CARTESIAN_POINT ( 'NONE',  ( 73.76535645333923696, 38.79159067395544014, 9.975000000000001421 ) ) ;
#4862=LINE ( 'NONE', #1294, #6940 ) ;
#4875=CARTESIAN_POINT ( 'NONE',  ( 70.26535645333922275, 38.79159067395544014, 7.600000000000002309 ) ) ;
#4882=AXIS2_PLACEMENT_3D ( 'NONE', #13952, #8050, #4554 ) ;
#4884=DIRECTION ( 'NONE',  ( -0.000000000000000000, -0.000000000000000000, 1.000000000000000000 ) ) ;
#4893=DIRECTION ( 'NONE',  ( -0.000000000000000000, 0.000000000000000000, 1.000000000000000000 ) ) ;
#4894=EDGE_CURVE ( 'NONE', #6169, #2150, #752, .T. ) ;
#4920=EDGE_LOOP ( 'NONE', ( #15154, #8510, #11524, #2524 ) ) ;
#4925=EDGE_LOOP ( 'NONE', ( #9126, #15617, #14053, #6671 ) ) ;
#4926=VERTEX_POINT ( 'NONE', #511 ) ;
#4929=ORIENTED_EDGE ( 'NONE', *, *, #1719, .T. ) ;
#4967=FACE_BOUND ( 'NONE', #14678, .T. ) ;
#4969=DIRECTION ( 'NONE',  ( -0.000000000000000000, -0.000000000000000000, 1.000000000000000000 ) ) ;
#4976=PRODUCT_DEFINITION ( 'UNKNOWN', '', #12817, #2843 ) ;
#4999=ORIENTED_EDGE ( 'NONE', *, *, #6638, .F. ) ;
#5024=ORIENTED_EDGE ( 'NONE', *, *, #14870, .F. ) ;
#5029=ADVANCED_FACE ( 'NONE', ( #10840 ), #8772, .F. ) ;
#5042=SURFACE_SIDE_STYLE ('',( #6312 ) ) ;
#5050=AXIS2_PLACEMENT_3D ( 'NONE', #6978, #10446, #875 ) ;
#5070=ORIENTED_EDGE ( 'NONE', *, *, #14922, .T. ) ;
#5072=FACE_OUTER_BOUND ( 'NONE', #9314, .T. ) ;
#5082=DIRECTION ( 'NONE',  ( -0.000000000000000000, -0.000000000000000000, -1.000000000000000000 ) ) ;
#5085=ADVANCED_FACE ( 'NONE', ( #9802 ), #14600, .F. ) ;
#5088=CIRCLE ( 'NONE', #7119, 1.700000000000000178 ) ;
#5095=DIRECTION ( 'NONE',  ( -0.000000000000000000, 0.000000000000000000, 1.000000000000000000 ) ) ;
#5103=FACE_OUTER_BOUND ( 'NONE', #15295, .T. ) ;
#5111=CARTESIAN_POINT ( 'NONE',  ( 122.5806775638430253, 45.00321902537314145, 9.975000000000001421 ) ) ;
#5119=DIRECTION ( 'NONE',  ( -0.000000000000000000, -0.000000000000000000, 1.000000000000000000 ) ) ;
#5121=FILL_AREA_STYLE_COLOUR ( '', #4090 ) ;
#5125=CARTESIAN_POINT ( 'NONE',  ( 172.5293059057019889, 61.25683321636181233, 10.00000000000000178 ) ) ;
#5138=CIRCLE ( 'NONE', #4882, 3.525000000000000355 ) ;
#5149=DIRECTION ( 'NONE',  ( 1.000000000000000000, 0.000000000000000000, 0.000000000000000000 ) ) ;
#5163=CIRCLE ( 'NONE', #10970, 1.700000000000007061 ) ;
#5173=ORIENTED_EDGE ( 'NONE', *, *, #3106, .F. ) ;
#5176=ORIENTED_EDGE ( 'NONE', *, *, #6734, .T. ) ;
#5182=LINE ( 'NONE', #656, #4285 ) ;
#5185=VECTOR ( 'NONE', #9258, 1000.000000000000114 ) ;
#5223=CARTESIAN_POINT ( 'NONE',  ( 186.1005832062958234, 72.46888774096882457, 5.000000000000000000 ) ) ;
#5229=VERTEX_POINT ( 'NONE', #3005 ) ;
#5234=LINE ( 'NONE', #9114, #3280 ) ;
#5244=DIRECTION ( 'NONE',  ( 1.000000000000000000, 0.000000000000000000, 0.000000000000000000 ) ) ;
#5264=CIRCLE ( 'NONE', #191, 325.5619230110239073 ) ;
#5270=CARTESIAN_POINT ( 'NONE',  ( -99.68324453533686835, 80.15913712344708131, 5.000000000000000000 ) ) ;
#5279=DIRECTION ( 'NONE',  ( -0.000000000000000000, -0.000000000000000000, 1.000000000000000000 ) ) ;
#5284=EDGE_LOOP ( 'NONE', ( #14887, #3856, #6417, #880 ) ) ;
#5302=EDGE_CURVE ( 'NONE', #12005, #13965, #8172, .T. ) ;
#5329=VERTEX_POINT ( 'NONE', #12855 ) ;
#5332=DIRECTION ( 'NONE',  ( 1.000000000000000000, 0.000000000000000000, 0.000000000000000000 ) ) ;
#5345=ORIENTED_EDGE ( 'NONE', *, *, #3154, .F. ) ;
#5379=DIRECTION ( 'NONE',  ( 1.000000000000000000, 0.000000000000000000, 0.000000000000000000 ) ) ;
#5383=AXIS2_PLACEMENT_3D ( 'NONE', #8691, #5279, #204 ) ;
#5421=EDGE_CURVE ( 'NONE', #10430, #6332, #601, .T. ) ;
#5442=CARTESIAN_POINT ( 'NONE',  ( 122.5806775638430253, 45.00321902537314145, 7.600000000000002309 ) ) ;
#5449=ORIENTED_EDGE ( 'NONE', *, *, #7116, .F. ) ;
#5453=EDGE_LOOP ( 'NONE', ( #4999, #10246 ) ) ;
#5459=ORIENTED_EDGE ( 'NONE', *, *, #622, .F. ) ;
#5496=CARTESIAN_POINT ( 'NONE',  ( 176.0293059057019889, 61.25683321636181233, 9.975000000000001421 ) ) ;
#5511=CARTESIAN_POINT ( 'NONE',  ( 19.11029453487719110, 40.04259805664093363, 10.00000000000000178 ) ) ;
#5520=DIRECTION ( 'NONE',  ( -0.000000000000000000, 0.000000000000000000, 1.000000000000000000 ) ) ;
#5527=FACE_OUTER_BOUND ( 'NONE', #6210, .T. ) ;
#5548=ORIENTED_EDGE ( 'NONE', *, *, #7733, .T. ) ;
#5551=VERTEX_POINT ( 'NONE', #5270 ) ;
#5561=VECTOR ( 'NONE', #15160, 1000.000000000000000 ) ;
#5626=DIRECTION ( 'NONE',  ( -0.000000000000000000, -0.000000000000000000, 1.000000000000000000 ) ) ;
#5631=FACE_OUTER_BOUND ( 'NONE', #7536, .T. ) ;
#5635=PRODUCT ( 'Upper Moving Shear Blade Bar', 'Upper Moving Shear Blade Bar', '', ( #10200 ) ) ;
#5641=ORIENTED_EDGE ( 'NONE', *, *, #13799, .T. ) ;
#5645=ORIENTED_EDGE ( 'NONE', *, *, #11620, .T. ) ;
#5646=CIRCLE ( 'NONE', #7173, 3.499999999999999556 ) ;
#5648=DIRECTION ( 'NONE',  ( -0.000000000000000000, -0.000000000000000000, 1.000000000000000000 ) ) ;
#5660=ADVANCED_FACE ( 'NONE', ( #3212, #4630, #5820, #9459, #9154, #9226, #10638 ), #8214, .T. ) ;
#5672=CARTESIAN_POINT ( 'NONE',  ( -111.2071507613730290, 58.10263819636593041, 10.00000000000000178 ) ) ;
#5676=CARTESIAN_POINT ( 'NONE',  ( 17.41029453487719181, 40.04259805664093363, 5.000000000000000000 ) ) ;
#5678=CARTESIAN_POINT ( 'NONE',  ( 73.76535645333923696, 38.79159067395544014, 7.600000000000002309 ) ) ;
#5681=DIRECTION ( 'NONE',  ( 1.000000000000000000, 0.000000000000000000, 0.000000000000000000 ) ) ;
#5726=EDGE_CURVE ( 'NONE', #14924, #15074, #5138, .T. ) ;
#5760=DIRECTION ( 'NONE',  ( 1.000000000000000000, 0.000000000000000000, 0.000000000000000000 ) ) ;
#5785=FACE_OUTER_BOUND ( 'NONE', #14833, .T. ) ;
#5807=ORIENTED_EDGE ( 'NONE', *, *, #11754, .T. ) ;
#5818=EDGE_CURVE ( 'NONE', #12823, #7872, #7970, .T. ) ;
#5820=FACE_BOUND ( 'NONE', #4542, .T. ) ;
#5821=CYLINDRICAL_SURFACE ( 'NONE', #11013, 1.700000000000007061 ) ;
#5831=CIRCLE ( 'NONE', #8899, 3.500000000000003109 ) ;
#5856=EDGE_CURVE ( 'NONE', #8789, #7454, #10697, .T. ) ;
#5859=FACE_OUTER_BOUND ( 'NONE', #8045, .T. ) ;
#5869=DIRECTION ( 'NONE',  ( 0.4630766004634062072, 0.8863182623094566503, 0.000000000000000000 ) ) ;
#5907=DIRECTION ( 'NONE',  ( -0.000000000000000000, -0.000000000000000000, 1.000000000000000000 ) ) ;
#5908=LINE ( 'NONE', #2195, #4216 ) ;
#5914=DIRECTION ( 'NONE',  ( -0.000000000000000000, -0.000000000000000000, 1.000000000000000000 ) ) ;
#5922=ORIENTED_EDGE ( 'NONE', *, *, #4004, .T. ) ;
#5928=EDGE_CURVE ( 'NONE', #256, #11858, #5646, .T. ) ;
#5939=APPLICATION_CONTEXT ( 'automotive_design' ) ;
#5940=DIRECTION ( 'NONE',  ( -0.9099397267342597129, -0.4147405137080060755, 0.000000000000000000 ) ) ;
#5964=ORIENTED_EDGE ( 'NONE', *, *, #6017, .T. ) ;
#5971=CIRCLE ( 'NONE', #14775, 1.699999999999993072 ) ;
#5984=FACE_OUTER_BOUND ( 'NONE', #14368, .T. ) ;
#5997=FACE_BOUND ( 'NONE', #8865, .T. ) ;
#6010=VERTEX_POINT ( 'NONE', #8978 ) ;
#6012=DIRECTION ( 'NONE',  ( -0.000000000000000000, -0.000000000000000000, 1.000000000000000000 ) ) ;
#6017=EDGE_CURVE ( 'NONE', #4350, #956, #15462, .T. ) ;
#6023=CIRCLE ( 'NONE', #6921, 3.500000000000003109 ) ;
#6025=ORIENTED_EDGE ( 'NONE', *, *, #938, .F. ) ;
#6036=LINE ( 'NONE', #12181, #1741 ) ;
#6057=VECTOR ( 'NONE', #10521, 1000.000000000000000 ) ;
#6061=EDGE_CURVE ( 'NONE', #158, #935, #6917, .T. ) ;
#6065=CARTESIAN_POINT ( 'NONE',  ( -85.27455057502459113, 65.19100426474074084, 10.00000000000000178 ) ) ;
#6068=CIRCLE ( 'NONE', #7081, 3.500000000000003109 ) ;
#6100=CARTESIAN_POINT ( 'NONE',  ( 70.26535645333922275, 38.79159067395544014, 10.00000000000000178 ) ) ;
#6101=FACE_OUTER_BOUND ( 'NONE', #14454, .T. ) ;
#6103=CARTESIAN_POINT ( 'NONE',  ( -38.32399788034579302, 48.72489408690345414, 10.00000000000000178 ) ) ;
#6127=FACE_OUTER_BOUND ( 'NONE', #1096, .T. ) ;
#6135=ORIENTED_EDGE ( 'NONE', *, *, #9243, .F. ) ;
#6138=ADVANCED_FACE ( 'NONE', ( #15026, #5103 ), #14719, .F. ) ;
#6148=VECTOR ( 'NONE', #11748, 1000.000000000000000 ) ;
#6165=AXIS2_PLACEMENT_3D ( 'NONE', #12431, #13772, #492 ) ;
#6169=VERTEX_POINT ( 'NONE', #4449 ) ;
#6206=DIRECTION ( 'NONE',  ( 1.000000000000000000, 0.000000000000000000, 0.000000000000000000 ) ) ;
#6210=EDGE_LOOP ( 'NONE', ( #749, #11082, #4167, #63 ) ) ;
#6217=DIRECTION ( 'NONE',  ( -0.000000000000000000, -0.000000000000000000, 1.000000000000000000 ) ) ;
#6219=DIRECTION ( 'NONE',  ( 1.000000000000000000, 0.000000000000000000, 0.000000000000000000 ) ) ;
#6234=DIRECTION ( 'NONE',  ( -0.000000000000000000, 0.000000000000000000, 1.000000000000000000 ) ) ;
#6258=EDGE_LOOP ( 'NONE', ( #11769, #447 ) ) ;
#6262=AXIS2_PLACEMENT_3D ( 'NONE', #2674, #5119, #7423 ) ;
#6263=LINE ( 'NONE', #13431, #8599 ) ;
#6297=FACE_OUTER_BOUND ( 'NONE', #2249, .T. ) ;
#6312=SURFACE_STYLE_FILL_AREA ( #7738 ) ;
#6332=VERTEX_POINT ( 'NONE', #11009 ) ;
#6340=EDGE_CURVE ( 'NONE', #1426, #12939, #6036, .T. ) ;
#6342=EDGE_LOOP ( 'NONE', ( #3706, #13735 ) ) ;
#6377=EDGE_CURVE ( 'NONE', #14684, #12005, #90, .T. ) ;
#6385=CARTESIAN_POINT ( 'NONE',  ( -86.97455057502459397, 65.19100426474074084, 5.000000000000000000 ) ) ;
#6402=AXIS2_PLACEMENT_3D ( 'NONE', #2184, #834, #3140 ) ;
#6403=CARTESIAN_POINT ( 'NONE',  ( 20.91029453487719181, 40.04259805664093363, 7.600000000000002309 ) ) ;
#6415=DIRECTION ( 'NONE',  ( 1.000000000000000000, 0.000000000000000000, 0.000000000000000000 ) ) ;
#6417=ORIENTED_EDGE ( 'NONE', *, *, #10292, .F. ) ;
#6425=ORIENTED_EDGE ( 'NONE', *, *, #1682, .F. ) ;
#6429=EDGE_LOOP ( 'NONE', ( #9400, #6425, #9897, #7688 ) ) ;
#6432=CIRCLE ( 'NONE', #847, 1.700000000000007061 ) ;
#6439=DIRECTION ( 'NONE',  ( -0.000000000000000000, 0.000000000000000000, 1.000000000000000000 ) ) ;
#6468=DIRECTION ( 'NONE',  ( -0.000000000000000000, -0.000000000000000000, 1.000000000000000000 ) ) ;
#6479=ADVANCED_FACE ( 'NONE', ( #4046 ), #11314, .T. ) ;
#6518=AXIS2_PLACEMENT_3D ( 'NONE', #14889, #8916, #3859 ) ;
#6523=CIRCLE ( 'NONE', #2724, 338.5619230110239641 ) ;
#6532=DIRECTION ( 'NONE',  ( -0.000000000000000000, -0.000000000000000000, 1.000000000000000000 ) ) ;
#6562=CARTESIAN_POINT ( 'NONE',  ( 120.8806775638430224, 45.00321902537314145, 5.000000000000000000 ) ) ;
#6568=VERTEX_POINT ( 'NONE', #13991 ) ;
#6583=CARTESIAN_POINT ( 'NONE',  ( 172.5293059057019889, 61.25683321636181233, 10.00000000000000178 ) ) ;
#6599=AXIS2_PLACEMENT_3D ( 'NONE', #3063, #13946, #6773 ) ;
#6620=DIRECTION ( 'NONE',  ( 1.000000000000000000, 0.000000000000000000, 0.000000000000000000 ) ) ;
#6623=AXIS2_PLACEMENT_3D ( 'NONE', #4013, #8847, #10984 ) ;
#6629=ORIENTED_EDGE ( 'NONE', *, *, #5726, .T. ) ;
#6638=EDGE_CURVE ( 'NONE', #2150, #12939, #2519, .T. ) ;
#6655=CARTESIAN_POINT ( 'NONE',  ( 122.5806775638430253, 45.00321902537314145, 7.600000000000002309 ) ) ;
#6667=FACE_OUTER_BOUND ( 'NONE', #6258, .T. ) ;
#6671=ORIENTED_EDGE ( 'NONE', *, *, #11293, .F. ) ;
#6675=CARTESIAN_POINT ( 'NONE',  ( -33.09899788034579871, 48.72489408690345414, 5.000000000000000000 ) ) ;
#6696=EDGE_CURVE ( 'NONE', #10652, #12061, #9588, .T. ) ;
#6706=VERTEX_POINT ( 'NONE', #6675 ) ;
#6713=VECTOR ( 'NONE', #9899, 1000.000000000000000 ) ;
#6720=EDGE_LOOP ( 'NONE', ( #12103, #7767, #7382, #1222 ) ) ;
#6723=DIRECTION ( 'NONE',  ( -0.000000000000000000, -0.000000000000000000, 1.000000000000000000 ) ) ;
#6734=EDGE_CURVE ( 'NONE', #14322, #7924, #9948, .T. ) ;
#6741=CARTESIAN_POINT ( 'NONE',  ( 71.96535645333923981, 38.79159067395544014, 5.000000000000000000 ) ) ;
#6760=CARTESIAN_POINT ( 'NONE',  ( 17.41029453487719181, 40.04259805664093363, 10.00000000000000178 ) ) ;
#6773=DIRECTION ( 'NONE',  ( -1.000000000000000000, 0.000000000000000000, -0.000000000000000000 ) ) ;
#6795=CYLINDRICAL_SURFACE ( 'NONE', #14895, 3.500000000000003109 ) ;
#6811=CARTESIAN_POINT ( 'NONE',  ( -85.27455057502459113, 65.19100426474074084, 10.00000000000000178 ) ) ;
#6817=ORIENTED_EDGE ( 'NONE', *, *, #13914, .F. ) ;
#6821=AXIS2_PLACEMENT_3D ( 'NONE', #14493, #5907, #7261 ) ;
#6826=ADVANCED_FACE ( 'NONE', ( #287 ), #4793, .F. ) ;
#6839=EDGE_CURVE ( 'NONE', #12197, #158, #8757, .T. ) ;
#6917=CIRCLE ( 'NONE', #6165, 3.500000000000003109 ) ;
#6921=AXIS2_PLACEMENT_3D ( 'NONE', #12677, #3372, #8132 ) ;
#6923=VECTOR ( 'NONE', #12926, 1000.000000000000000 ) ;
#6927=DIRECTION ( 'NONE',  ( 1.000000000000000000, 0.000000000000000000, 0.000000000000000000 ) ) ;
#6936=ORIENTED_EDGE ( 'NONE', *, *, #12619, .F. ) ;
#6940=VECTOR ( 'NONE', #13211, 1000.000000000000000 ) ;
#6969=CARTESIAN_POINT ( 'NONE',  ( 120.8806775638430224, 45.00321902537314145, 10.00000000000000178 ) ) ;
#6973=DIRECTION ( 'NONE',  ( -0.000000000000000000, -0.000000000000000000, 1.000000000000000000 ) ) ;
#6978=CARTESIAN_POINT ( 'NONE',  ( -85.27455057502459113, 65.19100426474074084, 7.600000000000002309 ) ) ;
#6980=DIRECTION ( 'NONE',  ( -0.000000000000000000, -0.000000000000000000, 1.000000000000000000 ) ) ;
#6997=EDGE_CURVE ( 'NONE', #14684, #457, #6068, .T. ) ;
#7007=ORIENTED_EDGE ( 'NONE', *, *, #5421, .T. ) ;
#7008=ORIENTED_EDGE ( 'NONE', *, *, #11583, .T. ) ;
#7028=AXIS2_PLACEMENT_3D ( 'NONE', #6811, #3405, #1029 ) ;
#7037=ADVANCED_FACE ( 'NONE', ( #12052 ), #7412, .F. ) ;
#7043=CARTESIAN_POINT ( 'NONE',  ( 172.5293059057019889, 61.25683321636181233, 9.975000000000001421 ) ) ;
#7051=AXIS2_PLACEMENT_3D ( 'NONE', #9024, #7690, #9980 ) ;
#7052=ADVANCED_FACE ( 'NONE', ( #342 ), #11352, .F. ) ;
#7071=ORIENTED_EDGE ( 'NONE', *, *, #5856, .T. ) ;
#7072=VECTOR ( 'NONE', #4969, 1000.000000000000000 ) ;
#7081=AXIS2_PLACEMENT_3D ( 'NONE', #11113, #266, #13387 ) ;
#7087=DIRECTION ( 'NONE',  ( 0.4630766004634062072, 0.8863182623094566503, 0.000000000000000000 ) ) ;
#7103=DIRECTION ( 'NONE',  ( 1.000000000000000000, 0.000000000000000000, 0.000000000000000000 ) ) ;
#7107=ORIENTED_EDGE ( 'NONE', *, *, #2859, .F. ) ;
#7116=EDGE_CURVE ( 'NONE', #6706, #2958, #5182, .T. ) ;
#7119=AXIS2_PLACEMENT_3D ( 'NONE', #1085, #10651, #9389 ) ;
#7128=ADVANCED_FACE ( 'NONE', ( #414 ), #8902, .F. ) ;
#7132=VERTEX_POINT ( 'NONE', #5496 ) ;
#7137=CARTESIAN_POINT ( 'NONE',  ( -86.97455057502459397, 65.19100426474074084, 7.600000000000002309 ) ) ;
#7142=DIRECTION ( 'NONE',  ( -1.000000000000000000, 0.000000000000000000, -0.000000000000000000 ) ) ;
#7144=CARTESIAN_POINT ( 'NONE',  ( -85.27455057502459113, 65.19100426474074084, 10.00000000000000178 ) ) ;
#7147=EDGE_LOOP ( 'NONE', ( #589, #12930, #9019, #5070 ) ) ;
#7162=CARTESIAN_POINT ( 'NONE',  ( 126.0806775638430253, 45.00321902537314145, 10.00000000000000178 ) ) ;
#7166=DIRECTION ( 'NONE',  ( -0.000000000000000000, -0.000000000000000000, -1.000000000000000000 ) ) ;
#7169=CARTESIAN_POINT ( 'NONE',  ( 66.76535645333922275, 38.79159067395544014, 9.975000000000001421 ) ) ;
#7173=AXIS2_PLACEMENT_3D ( 'NONE', #7479, #1226, #4708 ) ;
#7189=DIRECTION ( 'NONE',  ( -0.000000000000000000, -0.000000000000000000, 1.000000000000000000 ) ) ;
#7198=FACE_OUTER_BOUND ( 'NONE', #12216, .T. ) ;
#7210=ORIENTED_EDGE ( 'NONE', *, *, #3469, .F. ) ;
#7215=DIRECTION ( 'NONE',  ( 1.000000000000000000, 0.000000000000000000, 0.000000000000000000 ) ) ;
#7234=DIRECTION ( 'NONE',  ( -0.000000000000000000, -0.000000000000000000, 1.000000000000000000 ) ) ;
#7241=EDGE_LOOP ( 'NONE', ( #5173, #2181, #5548, #9764 ) ) ;
#7261=DIRECTION ( 'NONE',  ( 1.000000000000000000, 0.000000000000000000, 0.000000000000000000 ) ) ;
#7269=CARTESIAN_POINT ( 'NONE',  ( -88.77455057502459113, 65.19100426474074084, 9.975000000000001421 ) ) ;
#7277=AXIS2_PLACEMENT_3D ( 'NONE', #4752, #15548, #7142 ) ;
#7278=ORIENTED_EDGE ( 'NONE', *, *, #9098, .F. ) ;
#7291=CYLINDRICAL_SURFACE ( 'NONE', #8093, 3.500000000000003109 ) ;
#7311=CYLINDRICAL_SURFACE ( 'NONE', #9323, 1.700000000000000178 ) ;
#7325=DIRECTION ( 'NONE',  ( 1.000000000000000000, 0.000000000000000000, 0.000000000000000000 ) ) ;
#7327=ORIENTED_EDGE ( 'NONE', *, *, #3721, .T. ) ;
#7367=ORIENTED_EDGE ( 'NONE', *, *, #10292, .T. ) ;
#7371=ADVANCED_FACE ( 'NONE', ( #13364 ), #7311, .F. ) ;
#7373=VERTEX_POINT ( 'NONE', #1286 ) ;
#7382=ORIENTED_EDGE ( 'NONE', *, *, #12403, .T. ) ;
#7406=VERTEX_POINT ( 'NONE', #9591 ) ;
#7412=CYLINDRICAL_SURFACE ( 'NONE', #754, 1.700000000000007061 ) ;
#7423=DIRECTION ( 'NONE',  ( 1.000000000000000000, 0.000000000000000000, 0.000000000000000000 ) ) ;
#7431=ORIENTED_EDGE ( 'NONE', *, *, #3981, .F. ) ;
#7454=VERTEX_POINT ( 'NONE', #15 ) ;
#7479=CARTESIAN_POINT ( 'NONE',  ( 17.41029453487719181, 40.04259805664093363, 9.975000000000001421 ) ) ;
#7484=VECTOR ( 'NONE', #5648, 1000.000000000000000 ) ;
#7492=LINE ( 'NONE', #14962, #13425 ) ;
#7495=CARTESIAN_POINT ( 'NONE',  ( 20.91029453487719181, 40.04259805664093363, 9.975000000000001421 ) ) ;
#7515=EDGE_CURVE ( 'NONE', #828, #4926, #8070, .T. ) ;
#7525=CARTESIAN_POINT ( 'NONE',  ( 51.07686401294030532, 368.7106150007013525, 5.000000000000000000 ) ) ;
#7536=EDGE_LOOP ( 'NONE', ( #13813, #7967 ) ) ;
#7548=CARTESIAN_POINT ( 'NONE',  ( -83.57455057502457407, 65.19100426474074084, 7.600000000000002309 ) ) ;
#7581=DIRECTION ( 'NONE',  ( -0.000000000000000000, -0.000000000000000000, 1.000000000000000000 ) ) ;
#7594=DIRECTION ( 'NONE',  ( -0.000000000000000000, -0.000000000000000000, 1.000000000000000000 ) ) ;
#7598=DIRECTION ( 'NONE',  ( -0.000000000000000000, -0.000000000000000000, 1.000000000000000000 ) ) ;
#7605=ADVANCED_FACE ( 'NONE', ( #3900 ), #14855, .F. ) ;
#7609=CARTESIAN_POINT ( 'NONE',  ( 73.79035645333922844, 38.79159067395544014, 10.00000000000000178 ) ) ;
#7615=ORIENTED_EDGE ( 'NONE', *, *, #2102, .F. ) ;
#7646=DIRECTION ( 'NONE',  ( -0.000000000000000000, -0.000000000000000000, 1.000000000000000000 ) ) ;
#7688=ORIENTED_EDGE ( 'NONE', *, *, #1633, .T. ) ;
#7690=DIRECTION ( 'NONE',  ( 0.000000000000000000, 0.000000000000000000, -1.000000000000000000 ) ) ;
#7695=AXIS2_PLACEMENT_3D ( 'NONE', #9142, #12746, #15110 ) ;
#7699=CARTESIAN_POINT ( 'NONE',  ( 51.07686401294030532, 368.7106150007013525, 10.00000000000000178 ) ) ;
#7700=PLANE ( 'NONE',  #3937 ) ;
#7703=ADVANCED_FACE ( 'NONE', ( #11714 ), #9347, .F. ) ;
#7712=CARTESIAN_POINT ( 'NONE',  ( 20.93529453487719039, 40.04259805664093363, 10.00000000000000178 ) ) ;
#7720=CARTESIAN_POINT ( 'NONE',  ( 122.5806775638430253, 45.00321902537314145, 10.00000000000000178 ) ) ;
#7730=ORIENTED_EDGE ( 'NONE', *, *, #12505, .T. ) ;
#7733=EDGE_CURVE ( 'NONE', #13786, #7132, #4276, .T. ) ;
#7738=FILL_AREA_STYLE ('',( #5121 ) ) ;
#7752=VERTEX_POINT ( 'NONE', #13918 ) ;
#7753=DIRECTION ( 'NONE',  ( 1.000000000000000000, 0.000000000000000000, 0.000000000000000000 ) ) ;
#7756=DIRECTION ( 'NONE',  ( 1.000000000000000000, 0.000000000000000000, 0.000000000000000000 ) ) ;
#7767=ORIENTED_EDGE ( 'NONE', *, *, #5856, .F. ) ;
#7775=DIRECTION ( 'NONE',  ( 1.000000000000000000, 0.000000000000000000, 0.000000000000000000 ) ) ;
#7788=CARTESIAN_POINT ( 'NONE',  ( 70.26535645333922275, 38.79159067395544014, 10.00000000000000178 ) ) ;
#7792=ORIENTED_EDGE ( 'NONE', *, *, #12403, .F. ) ;
#7853=ORIENTED_EDGE ( 'NONE', *, *, #2189, .F. ) ;
#7855=CARTESIAN_POINT ( 'NONE',  ( -85.27455057502459113, 65.19100426474074084, 5.000000000000000000 ) ) ;
#7862=CARTESIAN_POINT ( 'NONE',  ( 19.11029453487719110, 40.04259805664093363, 7.600000000000002309 ) ) ;
#7872=VERTEX_POINT ( 'NONE', #6103 ) ;
#7875=ORIENTED_EDGE ( 'NONE', *, *, #1861, .T. ) ;
#7894=CARTESIAN_POINT ( 'NONE',  ( -83.57455057502457407, 65.19100426474074084, 5.000000000000000000 ) ) ;
#7924=VERTEX_POINT ( 'NONE', #7137 ) ;
#7952=DIRECTION ( 'NONE',  ( -0.000000000000000000, -0.000000000000000000, 1.000000000000000000 ) ) ;
#7957=ORIENTED_EDGE ( 'NONE', *, *, #13818, .F. ) ;
#7958=DIRECTION ( 'NONE',  ( -0.000000000000000000, -0.000000000000000000, 1.000000000000000000 ) ) ;
#7967=ORIENTED_EDGE ( 'NONE', *, *, #12504, .T. ) ;
#7970=LINE ( 'NONE', #4394, #6148 ) ;
#7978=ADVANCED_FACE ( 'NONE', ( #9654 ), #8625, .F. ) ;
#8045=EDGE_LOOP ( 'NONE', ( #10510, #7957, #13280, #143 ) ) ;
#8049=CIRCLE ( 'NONE', #1713, 3.500000000000003109 ) ;
#8050=DIRECTION ( 'NONE',  ( -0.000000000000000000, -0.000000000000000000, 1.000000000000000000 ) ) ;
#8058=DIRECTION ( 'NONE',  ( -0.000000000000000000, 0.000000000000000000, 1.000000000000000000 ) ) ;
#8059=CIRCLE ( 'NONE', #12558, 1.700000000000007061 ) ;
#8062=( NAMED_UNIT ( * ) PLANE_ANGLE_UNIT ( ) SI_UNIT ( $, .RADIAN. ) );
#8070=CIRCLE ( 'NONE', #13344, 1.700000000000007061 ) ;
#8072=CARTESIAN_POINT ( 'NONE',  ( 176.0543059057019661, 61.25683321636181233, 10.00000000000000178 ) ) ;
#8074=ADVANCED_FACE ( 'NONE', ( #540 ), #10409, .F. ) ;
#8085=DIRECTION ( 'NONE',  ( 1.000000000000000000, 0.000000000000000000, 0.000000000000000000 ) ) ;
#8087=ORIENTED_EDGE ( 'NONE', *, *, #2664, .T. ) ;
#8093=AXIS2_PLACEMENT_3D ( 'NONE', #15540, #3801, #7215 ) ;
#8104=CARTESIAN_POINT ( 'NONE',  ( 191.4922098844999425, 60.63967129342340456, 10.00000000000000178 ) ) ;
#8121=LINE ( 'NONE', #11737, #4651 ) ;
#8132=DIRECTION ( 'NONE',  ( 1.000000000000000000, 0.000000000000000000, 0.000000000000000000 ) ) ;
#8147=DIRECTION ( 'NONE',  ( 0.000000000000000000, 0.000000000000000000, 1.000000000000000000 ) ) ;
#8149=ADVANCED_FACE ( 'NONE', ( #1660 ), #14180, .F. ) ;
#8166=LINE ( 'NONE', #6969, #4553 ) ;
#8172=CIRCLE ( 'NONE', #12172, 3.525000000000000355 ) ;
#8174=ORIENTED_EDGE ( 'NONE', *, *, #7515, .T. ) ;
#8206=CARTESIAN_POINT ( 'NONE',  ( 15.71029453487719074, 40.04259805664093363, 5.000000000000000000 ) ) ;
#8214=PLANE ( 'NONE',  #6402 ) ;
#8233=AXIS2_PLACEMENT_3D ( 'NONE', #1275, #82, #15072 ) ;
#8244=LINE ( 'NONE', #4507, #13819 ) ;
#8246=VERTEX_POINT ( 'NONE', #8072 ) ;
#8272=CYLINDRICAL_SURFACE ( 'NONE', #13720, 325.5619230110239073 ) ;
#8288=EDGE_CURVE ( 'NONE', #4350, #13543, #7492, .T. ) ;
#8298=AXIS2_PLACEMENT_3D ( 'NONE', #47, #4884, #9703 ) ;
#8303=DIRECTION ( 'NONE',  ( -0.000000000000000000, 0.000000000000000000, 1.000000000000000000 ) ) ;
#8338=EDGE_LOOP ( 'NONE', ( #1463, #14858, #1171, #11402 ) ) ;
#8371=LINE ( 'NONE', #2506, #15615 ) ;
#8410=VERTEX_POINT ( 'NONE', #7894 ) ;
#8413=LINE ( 'NONE', #9504, #12861 ) ;
#8449=EDGE_CURVE ( 'NONE', #15218, #12185, #6023, .T. ) ;
#8496=AXIS2_PLACEMENT_3D ( 'NONE', #10368, #12489, #15162 ) ;
#8510=ORIENTED_EDGE ( 'NONE', *, *, #8288, .T. ) ;
#8553=FACE_OUTER_BOUND ( 'NONE', #5284, .T. ) ;
#8556=CIRCLE ( 'NONE', #3251, 3.525000000000000355 ) ;
#8557=CARTESIAN_POINT ( 'NONE',  ( -88.79955057502458260, 65.19100426474074084, 10.00000000000000178 ) ) ;
#8571=ORIENTED_EDGE ( 'NONE', *, *, #622, .T. ) ;
#8576=DIRECTION ( 'NONE',  ( -0.000000000000000000, -0.000000000000000000, 1.000000000000000000 ) ) ;
#8578=VECTOR ( 'NONE', #5869, 999.9999999999998863 ) ;
#8581=CARTESIAN_POINT ( 'NONE',  ( 51.07686401294030532, 368.7106150007013525, 5.000000000000000000 ) ) ;
#8599=VECTOR ( 'NONE', #9740, 1000.000000000000000 ) ;
#8604=DIRECTION ( 'NONE',  ( 1.000000000000000000, 0.000000000000000000, 0.000000000000000000 ) ) ;
#8606=DIRECTION ( 'NONE',  ( 1.000000000000000000, 0.000000000000000000, 0.000000000000000000 ) ) ;
#8625=CYLINDRICAL_SURFACE ( 'NONE', #2085, 1.700000000000000178 ) ;
#8636=EDGE_LOOP ( 'NONE', ( #11622, #5922, #12878, #175 ) ) ;
#8667=LINE ( 'NONE', #13459, #7484 ) ;
#8681=DIRECTION ( 'NONE',  ( -0.000000000000000000, -0.000000000000000000, 1.000000000000000000 ) ) ;
#8691=CARTESIAN_POINT ( 'NONE',  ( 17.41029453487719181, 40.04259805664093363, 10.00000000000000178 ) ) ;
#8692=AXIS2_PLACEMENT_3D ( 'NONE', #13151, #13390, #7103 ) ;
#8703=CIRCLE ( 'NONE', #13987, 3.525000000000000355 ) ;
#8720=DIRECTION ( 'NONE',  ( -0.000000000000000000, -0.000000000000000000, 1.000000000000000000 ) ) ;
#8730=DIRECTION ( 'NONE',  ( 1.000000000000000000, 0.000000000000000000, 0.000000000000000000 ) ) ;
#8735=ORIENTED_EDGE ( 'NONE', *, *, #6340, .T. ) ;
#8737=CIRCLE ( 'NONE', #13263, 3.525000000000000355 ) ;
#8746=DIRECTION ( 'NONE',  ( 1.000000000000000000, 0.000000000000000000, 0.000000000000000000 ) ) ;
#8756=CARTESIAN_POINT ( 'NONE',  ( 17.41029453487719181, 40.04259805664093363, 5.000000000000000000 ) ) ;
#8757=LINE ( 'NONE', #3863, #8836 ) ;
#8772=CYLINDRICAL_SURFACE ( 'NONE', #4105, 3.500000000000003109 ) ;
#8773=DIRECTION ( 'NONE',  ( 1.000000000000000000, 0.000000000000000000, 0.000000000000000000 ) ) ;
#8789=VERTEX_POINT ( 'NONE', #5678 ) ;
#8790=CARTESIAN_POINT ( 'NONE',  ( 172.5293059057019889, 61.25683321636181233, 5.000000000000000000 ) ) ;
#8820=EDGE_CURVE ( 'NONE', #15257, #7752, #753, .T. ) ;
#8836=VECTOR ( 'NONE', #12377, 1000.000000000000000 ) ;
#8847=DIRECTION ( 'NONE',  ( -0.000000000000000000, -0.000000000000000000, 1.000000000000000000 ) ) ;
#8865=EDGE_LOOP ( 'NONE', ( #8087, #5641 ) ) ;
#8871=EDGE_CURVE ( 'NONE', #7752, #15257, #4792, .T. ) ;
#8875=DIRECTION ( 'NONE',  ( -0.000000000000000000, -0.000000000000000000, 1.000000000000000000 ) ) ;
#8880=EDGE_CURVE ( 'NONE', #14396, #11858, #8371, .T. ) ;
#8883=CARTESIAN_POINT ( 'NONE',  ( 122.5806775638430253, 45.00321902537314145, 5.000000000000000000 ) ) ;
#8886=CONICAL_SURFACE ( 'NONE', #2059, 3.525000000000000355, 0.7853981633974482790 ) ;
#8888=DIRECTION ( 'NONE',  ( -0.000000000000000000, 0.000000000000000000, 1.000000000000000000 ) ) ;
#8899=AXIS2_PLACEMENT_3D ( 'NONE', #4646, #13891, #12698 ) ;
#8902=CYLINDRICAL_SURFACE ( 'NONE', #9597, 3.499999999999999556 ) ;
#8914=VERTEX_POINT ( 'NONE', #15481 ) ;
#8916=DIRECTION ( 'NONE',  ( -0.000000000000000000, -0.000000000000000000, 1.000000000000000000 ) ) ;
#8930=AXIS2_PLACEMENT_3D ( 'NONE', #5442, #675, #440 ) ;
#8936=ORIENTED_EDGE ( 'NONE', *, *, #2694, .F. ) ;
#8949=VERTEX_POINT ( 'NONE', #883 ) ;
#8959=CARTESIAN_POINT ( 'NONE',  ( -34.79899788034579444, 48.72489408690345414, 9.975000000000001421 ) ) ;
#8964=EDGE_CURVE ( 'NONE', #10355, #9645, #8413, .T. ) ;
#8972=VERTEX_POINT ( 'NONE', #10613 ) ;
#8978=CARTESIAN_POINT ( 'NONE',  ( 191.4922098844999425, 60.63967129342340456, 5.000000000000000000 ) ) ;
#9019=ORIENTED_EDGE ( 'NONE', *, *, #11245, .T. ) ;
#9024=CARTESIAN_POINT ( 'NONE',  ( 124.2806775638430281, 45.00321902537314145, 7.600000000000002309 ) ) ;
#9050=EDGE_CURVE ( 'NONE', #12061, #6010, #6263, .T. ) ;
#9091=ORIENTED_EDGE ( 'NONE', *, *, #6638, .T. ) ;
#9098=EDGE_CURVE ( 'NONE', #5229, #3979, #4042, .T. ) ;
#9102=LINE ( 'NONE', #11833, #14805 ) ;
#9107=ORIENTED_EDGE ( 'NONE', *, *, #6839, .T. ) ;
#9114=CARTESIAN_POINT ( 'NONE',  ( 71.96535645333923981, 38.79159067395544014, 10.00000000000000178 ) ) ;
#9126=ORIENTED_EDGE ( 'NONE', *, *, #12504, .F. ) ;
#9142=CARTESIAN_POINT ( 'NONE',  ( 17.41029453487719181, 40.04259805664093363, 7.600000000000002309 ) ) ;
#9149=FACE_OUTER_BOUND ( 'NONE', #1125, .T. ) ;
#9154=FACE_BOUND ( 'NONE', #12517, .T. ) ;
#9158=CLOSED_SHELL ( 'NONE', ( #7052, #11520, #11716, #4711, #11427, #7037, #8149, #120, #5085, #911, #13065, #7371, #11655, #1987, #4267, #2148, #2895, #9992, #11785, #12901, #6479, #13863, #5660, #2512, #13849, #12209, #3804, #15541, #418, #9482, #7605, #8074, #7978, #3550, #7128, #3645, #7703, #11947, #5029, #14259, #4110, #15355, #10455, #2950, #439, #6138, #13986, #6826 ) ) ;
#9175=EDGE_CURVE ( 'NONE', #828, #3731, #8166, .T. ) ;
#9200=VECTOR ( 'NONE', #3381, 1000.000000000000000 ) ;
#9206=ORIENTED_EDGE ( 'NONE', *, *, #12044, .F. ) ;
#9218=ORIENTED_EDGE ( 'NONE', *, *, #3919, .F. ) ;
#9221=EDGE_LOOP ( 'NONE', ( #14671, #10672 ) ) ;
#9226=FACE_BOUND ( 'NONE', #748, .T. ) ;
#9236=EDGE_LOOP ( 'NONE', ( #6025, #9206 ) ) ;
#9238=DIRECTION ( 'NONE',  ( 1.000000000000000000, 0.000000000000000000, 0.000000000000000000 ) ) ;
#9243=EDGE_CURVE ( 'NONE', #158, #15257, #507, .T. ) ;
#9248=VECTOR ( 'NONE', #14177, 1000.000000000000000 ) ;
#9258=DIRECTION ( 'NONE',  ( -0.7071067811865474617, 8.659560562354932858E-17, 0.7071067811865474617 ) ) ;
#9267=DIRECTION ( 'NONE',  ( 1.000000000000000000, 0.000000000000000000, 0.000000000000000000 ) ) ;
#9274=EDGE_CURVE ( 'NONE', #7454, #14684, #1554, .T. ) ;
#9301=ORIENTED_EDGE ( 'NONE', *, *, #8871, .F. ) ;
#9314=EDGE_LOOP ( 'NONE', ( #11871, #7875 ) ) ;
#9315=DIRECTION ( 'NONE',  ( -0.000000000000000000, -0.000000000000000000, 1.000000000000000000 ) ) ;
#9316=ORIENTED_EDGE ( 'NONE', *, *, #6340, .F. ) ;
#9323=AXIS2_PLACEMENT_3D ( 'NONE', #2562, #10939, #9512 ) ;
#9347=CYLINDRICAL_SURFACE ( 'NONE', #11104, 1.700000000000007061 ) ;
#9349=AXIS2_PLACEMENT_3D ( 'NONE', #6655, #7598, #8773 ) ;
#9387=LINE ( 'NONE', #15210, #6923 ) ;
#9389=DIRECTION ( 'NONE',  ( 1.000000000000000000, 0.000000000000000000, 0.000000000000000000 ) ) ;
#9400=ORIENTED_EDGE ( 'NONE', *, *, #5818, .F. ) ;
#9425=CARTESIAN_POINT ( 'NONE',  ( 126.0806775638430253, 45.00321902537314145, 7.600000000000002309 ) ) ;
#9428=ORIENTED_EDGE ( 'NONE', *, *, #13719, .T. ) ;
#9459=FACE_BOUND ( 'NONE', #3732, .T. ) ;
#9465=VECTOR ( 'NONE', #803, 1000.000000000000000 ) ;
#9480=ORIENTED_EDGE ( 'NONE', *, *, #6061, .F. ) ;
#9482=ADVANCED_FACE ( 'NONE', ( #15115, #9149 ), #13869, .F. ) ;
#9504=CARTESIAN_POINT ( 'NONE',  ( -36.49899788034579018, 48.72489408690345414, 10.00000000000000178 ) ) ;
#9512=DIRECTION ( 'NONE',  ( 1.000000000000000000, 0.000000000000000000, 0.000000000000000000 ) ) ;
#9517=CARTESIAN_POINT ( 'NONE',  ( -99.68324453533686835, 80.15913712344708131, 10.00000000000000178 ) ) ;
#9522=EDGE_CURVE ( 'NONE', #13999, #13543, #5, .T. ) ;
#9535=CARTESIAN_POINT ( 'NONE',  ( -38.29899788034579444, 48.72489408690345414, 10.00000000000000178 ) ) ;
#9540=DIRECTION ( 'NONE',  ( -0.000000000000000000, -0.000000000000000000, 1.000000000000000000 ) ) ;
#9582=ORIENTED_EDGE ( 'NONE', *, *, #14030, .F. ) ;
#9588=CIRCLE ( 'NONE', #14357, 338.5619230110239641 ) ;
#9591=CARTESIAN_POINT ( 'NONE',  ( 71.96535645333923981, 38.79159067395544014, 7.600000000000002309 ) ) ;
#9597=AXIS2_PLACEMENT_3D ( 'NONE', #15028, #4215, #14950 ) ;
#9602=CARTESIAN_POINT ( 'NONE',  ( 51.07686401294030532, 368.7106150007013525, 10.00000000000000178 ) ) ;
#9610=CIRCLE ( 'NONE', #14869, 1.700000000000007061 ) ;
#9635=DIRECTION ( 'NONE',  ( 0.7071067811864983899, 0.000000000000000000, 0.7071067811865966446 ) ) ;
#9645=VERTEX_POINT ( 'NONE', #2558 ) ;
#9651=ORIENTED_EDGE ( 'NONE', *, *, #6734, .F. ) ;
#9653=CARTESIAN_POINT ( 'NONE',  ( 17.41029453487719181, 40.04259805664093363, 9.975000000000001421 ) ) ;
#9654=FACE_OUTER_BOUND ( 'NONE', #13438, .T. ) ;
#9659=ORIENTED_EDGE ( 'NONE', *, *, #2387, .T. ) ;
#9700=DIRECTION ( 'NONE',  ( -0.000000000000000000, -0.000000000000000000, 1.000000000000000000 ) ) ;
#9703=DIRECTION ( 'NONE',  ( 1.000000000000000000, 0.000000000000000000, 0.000000000000000000 ) ) ;
#9707=EDGE_CURVE ( 'NONE', #14322, #8410, #11638, .T. ) ;
#9736=PLANE ( 'NONE',  #7277 ) ;
#9740=DIRECTION ( 'NONE',  ( -0.000000000000000000, -0.000000000000000000, -1.000000000000000000 ) ) ;
#9742=VERTEX_POINT ( 'NONE', #11542 ) ;
#9743=ORIENTED_EDGE ( 'NONE', *, *, #1633, .F. ) ;
#9747=DIRECTION ( 'NONE',  ( -0.7071067811864983899, 8.659560562354331352E-17, 0.7071067811865966446 ) ) ;
#9749=VECTOR ( 'NONE', #9635, 1000.000000000000000 ) ;
#9753=EDGE_LOOP ( 'NONE', ( #2074, #5645, #15466, #10846 ) ) ;
#9761=ORIENTED_EDGE ( 'NONE', *, *, #5421, .F. ) ;
#9764=ORIENTED_EDGE ( 'NONE', *, *, #4649, .T. ) ;
#9780=CARTESIAN_POINT ( 'NONE',  ( 122.5806775638430253, 45.00321902537314145, 10.00000000000000178 ) ) ;
#9783=CARTESIAN_POINT ( 'NONE',  ( 70.26535645333922275, 38.79159067395544014, 10.00000000000000178 ) ) ;
#9785=CARTESIAN_POINT ( 'NONE',  ( -34.79899788034579444, 48.72489408690345414, 5.000000000000000000 ) ) ;
#9802=FACE_OUTER_BOUND ( 'NONE', #8636, .T. ) ;
#9844=AXIS2_PLACEMENT_3D ( 'NONE', #4433, #15084, #9267 ) ;
#9856=CIRCLE ( 'NONE', #15118, 3.525000000000000355 ) ;
#9859=CARTESIAN_POINT ( 'NONE',  ( -105.7032403413611092, 68.63699971342413164, 10.00000000000000178 ) ) ;
#9865=DIRECTION ( 'NONE',  ( -0.7071067811864983899, 8.659560562354331352E-17, 0.7071067811865966446 ) ) ;
#9870=SURFACE_STYLE_USAGE ( .BOTH. , #5042 ) ;
#9897=ORIENTED_EDGE ( 'NONE', *, *, #4021, .T. ) ;
#9899=DIRECTION ( 'NONE',  ( -0.000000000000000000, -0.000000000000000000, 1.000000000000000000 ) ) ;
#9927=EDGE_CURVE ( 'NONE', #15218, #4350, #12013, .T. ) ;
#9948=LINE ( 'NONE', #1476, #7072 ) ;
#9950=AXIS2_PLACEMENT_3D ( 'NONE', #4875, #109, #2658 ) ;
#9962=EDGE_LOOP ( 'NONE', ( #9651, #2974, #14365, #15493 ) ) ;
#9974=ORIENTED_EDGE ( 'NONE', *, *, #4894, .T. ) ;
#9976=FACE_OUTER_BOUND ( 'NONE', #7241, .T. ) ;
#9980=DIRECTION ( 'NONE',  ( -1.000000000000000000, 0.000000000000000000, -0.000000000000000000 ) ) ;
#9992=ADVANCED_FACE ( 'NONE', ( #372 ), #6795, .F. ) ;
#10015=FACE_OUTER_BOUND ( 'NONE', #7147, .T. ) ;
#10046=CYLINDRICAL_SURFACE ( 'NONE', #15296, 3.500000000000003109 ) ;
#10048=AXIS2_PLACEMENT_3D ( 'NONE', #8790, #3962, #2711 ) ;
#10084=CARTESIAN_POINT ( 'NONE',  ( 172.5293059057019889, 61.25683321636181233, 10.00000000000000178 ) ) ;
#10105=VECTOR ( 'NONE', #9865, 1000.000000000000000 ) ;
#10125=CARTESIAN_POINT ( 'NONE',  ( 17.41029453487719181, 40.04259805664093363, 7.600000000000002309 ) ) ;
#10170=ORIENTED_EDGE ( 'NONE', *, *, #3106, .T. ) ;
#10200=PRODUCT_CONTEXT ( 'NONE', #5939, 'mechanical' ) ;
#10202=AXIS2_PLACEMENT_3D ( 'NONE', #1341, #2776, #12085 ) ;
#10211=CYLINDRICAL_SURFACE ( 'NONE', #4237, 1.700000000000007061 ) ;
#10213=AXIS2_PLACEMENT_3D ( 'NONE', #1781, #10316, #12824 ) ;
#10214=ORIENTED_EDGE ( 'NONE', *, *, #5818, .T. ) ;
#10225=LINE ( 'NONE', #13604, #454 ) ;
#10229=ORIENTED_EDGE ( 'NONE', *, *, #11167, .T. ) ;
#10239=AXIS2_PLACEMENT_3D ( 'NONE', #5672, #10490, #12843 ) ;
#10246=ORIENTED_EDGE ( 'NONE', *, *, #11651, .F. ) ;
#10252=CARTESIAN_POINT ( 'NONE',  ( -38.29899788034578734, 48.72489408690345414, 9.975000000000001421 ) ) ;
#10281=CARTESIAN_POINT ( 'NONE',  ( 174.2293059057019775, 61.25683321636181233, 7.600000000000002309 ) ) ;
#10288=AXIS2_PLACEMENT_3D ( 'NONE', #5676, #10804, #15593 ) ;
#10290=FACE_BOUND ( 'NONE', #5453, .T. ) ;
#10292=EDGE_CURVE ( 'NONE', #12061, #4465, #4485, .T. ) ;
#10295=CIRCLE ( 'NONE', #6518, 1.700000000000007061 ) ;
#10302=CARTESIAN_POINT ( 'NONE',  ( 70.26535645333922275, 38.79159067395544014, 7.600000000000002309 ) ) ;
#10316=DIRECTION ( 'NONE',  ( -0.000000000000000000, -0.000000000000000000, 1.000000000000000000 ) ) ;
#10343=CARTESIAN_POINT ( 'NONE',  ( 70.26535645333922275, 38.79159067395544014, 9.975000000000001421 ) ) ;
#10355=VERTEX_POINT ( 'NONE', #52 ) ;
#10368=CARTESIAN_POINT ( 'NONE',  ( 17.41029453487719181, 40.04259805664093363, 10.00000000000000178 ) ) ;
#10409=CONICAL_SURFACE ( 'NONE', #11919, 3.525000000000000355, 0.7853981633975176679 ) ;
#10430=VERTEX_POINT ( 'NONE', #1393 ) ;
#10432=SHAPE_DEFINITION_REPRESENTATION ( #1706, #556 ) ;
#10438=DIRECTION ( 'NONE',  ( 1.000000000000000000, 0.000000000000000000, 0.000000000000000000 ) ) ;
#10442=ORIENTED_EDGE ( 'NONE', *, *, #6061, .T. ) ;
#10444=DIRECTION ( 'NONE',  ( -0.000000000000000000, 0.000000000000000000, 1.000000000000000000 ) ) ;
#10446=DIRECTION ( 'NONE',  ( -0.000000000000000000, -0.000000000000000000, 1.000000000000000000 ) ) ;
#10454=ORIENTED_EDGE ( 'NONE', *, *, #3981, .T. ) ;
#10455=ADVANCED_FACE ( 'NONE', ( #3621 ), #2437, .F. ) ;
#10490=DIRECTION ( 'NONE',  ( -0.8863182623094566503, 0.4630766004634062072, 0.000000000000000000 ) ) ;
#10493=DIRECTION ( 'NONE',  ( 1.000000000000000000, 0.000000000000000000, 0.000000000000000000 ) ) ;
#10509=DIRECTION ( 'NONE',  ( -0.000000000000000000, -0.000000000000000000, 1.000000000000000000 ) ) ;
#10510=ORIENTED_EDGE ( 'NONE', *, *, #9175, .F. ) ;
#10515=LINE ( 'NONE', #11707, #14566 ) ;
#10521=DIRECTION ( 'NONE',  ( -0.000000000000000000, -0.000000000000000000, 1.000000000000000000 ) ) ;
#10531=AXIS2_PLACEMENT_3D ( 'NONE', #3219, #12845, #10493 ) ;
#10540=CONICAL_SURFACE ( 'NONE', #8298, 3.525000000000000355, 0.7853981633973787790 ) ;
#10544=DIRECTION ( 'NONE',  ( -0.000000000000000000, -0.000000000000000000, 1.000000000000000000 ) ) ;
#10566=CARTESIAN_POINT ( 'NONE',  ( 70.26535645333922275, 38.79159067395544014, 5.000000000000000000 ) ) ;
#10584=ORIENTED_EDGE ( 'NONE', *, *, #1682, .T. ) ;
#10609=CIRCLE ( 'NONE', #3295, 3.500000000000003109 ) ;
#10613=CARTESIAN_POINT ( 'NONE',  ( -81.77455057502459113, 65.19100426474074084, 7.600000000000002309 ) ) ;
#10628=DIRECTION ( 'NONE',  ( -1.000000000000000000, 0.000000000000000000, -0.000000000000000000 ) ) ;
#10638=FACE_OUTER_BOUND ( 'NONE', #13562, .T. ) ;
#10651=DIRECTION ( 'NONE',  ( -0.000000000000000000, -0.000000000000000000, 1.000000000000000000 ) ) ;
#10652=VERTEX_POINT ( 'NONE', #738 ) ;
#10672=ORIENTED_EDGE ( 'NONE', *, *, #11322, .T. ) ;
#10680=CARTESIAN_POINT ( 'NONE',  ( 17.41029453487719181, 40.04259805664093363, 10.00000000000000178 ) ) ;
#10697=CIRCLE ( 'NONE', #9950, 3.500000000000003109 ) ;
#10716=CIRCLE ( 'NONE', #14224, 3.525000000000000355 ) ;
#10730=EDGE_CURVE ( 'NONE', #12185, #956, #14313, .T. ) ;
#10750=ORIENTED_EDGE ( 'NONE', *, *, #9707, .T. ) ;
#10752=CYLINDRICAL_SURFACE ( 'NONE', #1974, 1.700000000000007061 ) ;
#10778=EDGE_CURVE ( 'NONE', #11836, #4465, #11409, .T. ) ;
#10788=ORIENTED_EDGE ( 'NONE', *, *, #4004, .F. ) ;
#10804=DIRECTION ( 'NONE',  ( -0.000000000000000000, 0.000000000000000000, 1.000000000000000000 ) ) ;
#10813=ORIENTED_EDGE ( 'NONE', *, *, #11767, .F. ) ;
#10814=DIRECTION ( 'NONE',  ( -0.000000000000000000, -0.000000000000000000, 1.000000000000000000 ) ) ;
#10816=CARTESIAN_POINT ( 'NONE',  ( -85.27455057502459113, 65.19100426474074084, 7.600000000000002309 ) ) ;
#10818=FACE_OUTER_BOUND ( 'NONE', #1726, .T. ) ;
#10839=EDGE_LOOP ( 'NONE', ( #9301, #1981 ) ) ;
#10840=FACE_OUTER_BOUND ( 'NONE', #6720, .T. ) ;
#10841=DIRECTION ( 'NONE',  ( -0.000000000000000000, -0.000000000000000000, 1.000000000000000000 ) ) ;
#10846=ORIENTED_EDGE ( 'NONE', *, *, #9050, .F. ) ;
#10869=FACE_OUTER_BOUND ( 'NONE', #11217, .T. ) ;
#10883=DIRECTION ( 'NONE',  ( -0.000000000000000000, -0.000000000000000000, 1.000000000000000000 ) ) ;
#10901=AXIS2_PLACEMENT_3D ( 'NONE', #1472, #8681, #13475 ) ;
#10929=DIRECTION ( 'NONE',  ( -0.000000000000000000, -0.000000000000000000, 1.000000000000000000 ) ) ;
#10937=CARTESIAN_POINT ( 'NONE',  ( 66.74035645333923128, 38.79159067395544014, 10.00000000000000178 ) ) ;
#10939=DIRECTION ( 'NONE',  ( -0.000000000000000000, -0.000000000000000000, 1.000000000000000000 ) ) ;
#10954=ORIENTED_EDGE ( 'NONE', *, *, #2433, .F. ) ;
#10967=CARTESIAN_POINT ( 'NONE',  ( 169.0043059057019832, 61.25683321636181233, 10.00000000000000178 ) ) ;
#10970=AXIS2_PLACEMENT_3D ( 'NONE', #12115, #4777, #11890 ) ;
#10984=DIRECTION ( 'NONE',  ( 1.000000000000000000, 0.000000000000000000, 0.000000000000000000 ) ) ;
#10995=CIRCLE ( 'NONE', #2671, 3.525000000000000355 ) ;
#10999=CARTESIAN_POINT ( 'NONE',  ( 186.1005832062958234, 72.46888774096882457, 10.00000000000000178 ) ) ;
#11009=CARTESIAN_POINT ( 'NONE',  ( -38.29899788034579444, 48.72489408690345414, 7.600000000000002309 ) ) ;
#11013=AXIS2_PLACEMENT_3D ( 'NONE', #6065, #10883, #38 ) ;
#11032=LINE ( 'NONE', #9859, #2391 ) ;
#11040=ORIENTED_EDGE ( 'NONE', *, *, #6696, .T. ) ;
#11049=EDGE_CURVE ( 'NONE', #10652, #11836, #1118, .T. ) ;
#11056=ORIENTED_EDGE ( 'NONE', *, *, #1604, .T. ) ;
#11082=ORIENTED_EDGE ( 'NONE', *, *, #13719, .F. ) ;
#11104=AXIS2_PLACEMENT_3D ( 'NONE', #12721, #6980, #3257 ) ;
#11113=CARTESIAN_POINT ( 'NONE',  ( 70.26535645333922275, 38.79159067395544014, 9.975000000000001421 ) ) ;
#11135=AXIS2_PLACEMENT_3D ( 'NONE', #7043, #15383, #13015 ) ;
#11142=FACE_OUTER_BOUND ( 'NONE', #11523, .T. ) ;
#11150=CARTESIAN_POINT ( 'NONE',  ( 70.26535645333922275, 38.79159067395544014, 10.00000000000000178 ) ) ;
#11167=EDGE_CURVE ( 'NONE', #4465, #11247, #1507, .T. ) ;
#11201=DIRECTION ( 'NONE',  ( 1.000000000000000000, 0.000000000000000000, 0.000000000000000000 ) ) ;
#11217=EDGE_LOOP ( 'NONE', ( #4031, #1937, #2451, #3224 ) ) ;
#11222=CARTESIAN_POINT ( 'NONE',  ( -85.27455057502459113, 65.19100426474074084, 10.00000000000000178 ) ) ;
#11231=CARTESIAN_POINT ( 'NONE',  ( 73.76535645333923696, 38.79159067395544014, 10.00000000000000178 ) ) ;
#11236=CARTESIAN_POINT ( 'NONE',  ( -85.27455057502459113, 65.19100426474074084, 10.00000000000000178 ) ) ;
#11245=EDGE_CURVE ( 'NONE', #457, #13965, #9387, .T. ) ;
#11247=VERTEX_POINT ( 'NONE', #5223 ) ;
#11251=DIRECTION ( 'NONE',  ( 1.000000000000000000, 0.000000000000000000, 0.000000000000000000 ) ) ;
#11293=EDGE_CURVE ( 'NONE', #13094, #256, #4032, .T. ) ;
#11314=CYLINDRICAL_SURFACE ( 'NONE', #4007, 338.5619230110239641 ) ;
#11322=EDGE_CURVE ( 'NONE', #8914, #3938, #6432, .T. ) ;
#11341=DIRECTION ( 'NONE',  ( -0.000000000000000000, -0.000000000000000000, 1.000000000000000000 ) ) ;
#11352=CONICAL_SURFACE ( 'NONE', #13359, 3.525000000000000355, 0.7853981633973787790 ) ;
#11363=AXIS2_PLACEMENT_3D ( 'NONE', #452, #4103, #6415 ) ;
#11376=DIRECTION ( 'NONE',  ( 1.000000000000000000, 0.000000000000000000, 0.000000000000000000 ) ) ;
#11391=DIRECTION ( 'NONE',  ( 1.000000000000000000, 0.000000000000000000, 0.000000000000000000 ) ) ;
#11402=ORIENTED_EDGE ( 'NONE', *, *, #11245, .F. ) ;
#11403=DIRECTION ( 'NONE',  ( -0.000000000000000000, -0.000000000000000000, 1.000000000000000000 ) ) ;
#11405=DIRECTION ( 'NONE',  ( 0.7071067811865474617, 0.000000000000000000, 0.7071067811865474617 ) ) ;
#11409=CIRCLE ( 'NONE', #1816, 325.5619230110239073 ) ;
#11427=ADVANCED_FACE ( 'NONE', ( #5984 ), #14416, .F. ) ;
#11458=ORIENTED_EDGE ( 'NONE', *, *, #9927, .F. ) ;
#11464=DIRECTION ( 'NONE',  ( -0.000000000000000000, 0.000000000000000000, 1.000000000000000000 ) ) ;
#11471=ORIENTED_EDGE ( 'NONE', *, *, #2664, .F. ) ;
#11474=AXIS2_PLACEMENT_3D ( 'NONE', #11662, #10544, #2096 ) ;
#11477=LINE ( 'NONE', #14850, #13872 ) ;
#11508=CONICAL_SURFACE ( 'NONE', #8496, 3.525000000000000355, 0.7853981633974482790 ) ;
#11520=ADVANCED_FACE ( 'NONE', ( #6297 ), #4072, .F. ) ;
#11523=EDGE_LOOP ( 'NONE', ( #10954, #15544, #1553, #5449 ) ) ;
#11524=ORIENTED_EDGE ( 'NONE', *, *, #11734, .T. ) ;
#11542=CARTESIAN_POINT ( 'NONE',  ( -105.7032403413611661, 68.63699971342407480, 5.000000000000000000 ) ) ;
#11547=DIRECTION ( 'NONE',  ( -1.000000000000000000, 0.000000000000000000, -0.000000000000000000 ) ) ;
#11555=( GEOMETRIC_REPRESENTATION_CONTEXT ( 3 ) GLOBAL_UNCERTAINTY_ASSIGNED_CONTEXT ( ( #3426 ) ) GLOBAL_UNIT_ASSIGNED_CONTEXT ( ( #15053, #8062, #4327 ) ) REPRESENTATION_CONTEXT ( 'NONE', 'WORKASPACE' ) );
#11566=CIRCLE ( 'NONE', #4750, 3.500000000000003109 ) ;
#11583=EDGE_CURVE ( 'NONE', #8246, #1098, #10716, .T. ) ;
#11588=EDGE_CURVE ( 'NONE', #10430, #5329, #270, .T. ) ;
#11594=PLANE ( 'NONE',  #10239 ) ;
#11607=DIRECTION ( 'NONE',  ( 1.000000000000000000, 0.000000000000000000, 0.000000000000000000 ) ) ;
#11608=DIRECTION ( 'NONE',  ( 1.000000000000000000, 0.000000000000000000, 0.000000000000000000 ) ) ;
#11620=EDGE_CURVE ( 'NONE', #10652, #9742, #11032, .T. ) ;
#11622=ORIENTED_EDGE ( 'NONE', *, *, #11322, .F. ) ;
#11638=CIRCLE ( 'NONE', #4561, 1.700000000000007061 ) ;
#11651=EDGE_CURVE ( 'NONE', #12939, #2150, #12215, .T. ) ;
#11655=ADVANCED_FACE ( 'NONE', ( #4457 ), #13221, .F. ) ;
#11662=CARTESIAN_POINT ( 'NONE',  ( -34.79899788034579444, 48.72489408690345414, 7.600000000000002309 ) ) ;
#11669=ORIENTED_EDGE ( 'NONE', *, *, #13656, .F. ) ;
#11682=FACE_OUTER_BOUND ( 'NONE', #1859, .T. ) ;
#11684=SHAPE_REPRESENTATION_RELATIONSHIP ( 'NONE' , 'NONE' ,  #556, #3584 ) ;
#11689=DIRECTION ( 'NONE',  ( 1.000000000000000000, 0.000000000000000000, 0.000000000000000000 ) ) ;
#11704=FACE_OUTER_BOUND ( 'NONE', #11976, .T. ) ;
#11707=CARTESIAN_POINT ( 'NONE',  ( 169.0043059057019832, 61.25683321636181233, 10.00000000000000178 ) ) ;
#11714=FACE_OUTER_BOUND ( 'NONE', #3448, .T. ) ;
#11716=ADVANCED_FACE ( 'NONE', ( #4543 ), #2975, .F. ) ;
#11734=EDGE_CURVE ( 'NONE', #13543, #13999, #8703, .T. ) ;
#11737=CARTESIAN_POINT ( 'NONE',  ( -99.68324453533686835, 80.15913712344708131, 10.00000000000000178 ) ) ;
#11748=DIRECTION ( 'NONE',  ( -0.7071067811865965336, 8.659560562355533132E-17, 0.7071067811864985009 ) ) ;
#11754=EDGE_CURVE ( 'NONE', #6332, #10430, #872, .T. ) ;
#11764=CARTESIAN_POINT ( 'NONE',  ( -34.79899788034579444, 48.72489408690345414, 7.600000000000002309 ) ) ;
#11767=EDGE_CURVE ( 'NONE', #11836, #5551, #8121, .T. ) ;
#11769=ORIENTED_EDGE ( 'NONE', *, *, #2189, .T. ) ;
#11785=ADVANCED_FACE ( 'NONE', ( #1139 ), #8272, .F. ) ;
#11806=EDGE_CURVE ( 'NONE', #935, #7752, #4862, .T. ) ;
#11817=CIRCLE ( 'NONE', #10048, 1.700000000000007061 ) ;
#11833=CARTESIAN_POINT ( 'NONE',  ( 181.4384305232223369, 82.69763993231136112, 5.000000000000000000 ) ) ;
#11836=VERTEX_POINT ( 'NONE', #9517 ) ;
#11841=VECTOR ( 'NONE', #9747, 1000.000000000000000 ) ;
#11844=EDGE_CURVE ( 'NONE', #3979, #5229, #5163, .T. ) ;
#11847=CONICAL_SURFACE ( 'NONE', #7028, 3.525000000000000355, 0.7853981633973787790 ) ;
#11858=VERTEX_POINT ( 'NONE', #2335 ) ;
#11871=ORIENTED_EDGE ( 'NONE', *, *, #15290, .T. ) ;
#11878=ORIENTED_EDGE ( 'NONE', *, *, #13818, .T. ) ;
#11890=DIRECTION ( 'NONE',  ( 1.000000000000000000, 0.000000000000000000, 0.000000000000000000 ) ) ;
#11914=ORIENTED_EDGE ( 'NONE', *, *, #3154, .T. ) ;
#11919=AXIS2_PLACEMENT_3D ( 'NONE', #1420, #4177, #5379 ) ;
#11936=DIRECTION ( 'NONE',  ( 1.000000000000000000, 0.000000000000000000, 0.000000000000000000 ) ) ;
#11947=ADVANCED_FACE ( 'NONE', ( #2487, #6127 ), #2172, .F. ) ;
#11958=AXIS2_PLACEMENT_3D ( 'NONE', #13852, #3047, #3914 ) ;
#11968=VERTEX_POINT ( 'NONE', #7548 ) ;
#11976=EDGE_LOOP ( 'NONE', ( #6135, #13047, #2237, #14818 ) ) ;
#12005=VERTEX_POINT ( 'NONE', #3749 ) ;
#12013=LINE ( 'NONE', #1180, #2307 ) ;
#12044=EDGE_CURVE ( 'NONE', #9645, #2958, #2141, .T. ) ;
#12052=FACE_OUTER_BOUND ( 'NONE', #1274, .T. ) ;
#12056=VECTOR ( 'NONE', #3331, 1000.000000000000000 ) ;
#12058=DIRECTION ( 'NONE',  ( 1.000000000000000000, 0.000000000000000000, 0.000000000000000000 ) ) ;
#12061=VERTEX_POINT ( 'NONE', #8104 ) ;
#12069=CARTESIAN_POINT ( 'NONE',  ( 0.000000000000000000, 0.000000000000000000, 5.000000000000000000 ) ) ;
#12085=DIRECTION ( 'NONE',  ( 1.000000000000000000, 0.000000000000000000, 0.000000000000000000 ) ) ;
#12089=DIRECTION ( 'NONE',  ( 1.000000000000000000, 0.000000000000000000, 0.000000000000000000 ) ) ;
#12103=ORIENTED_EDGE ( 'NONE', *, *, #9274, .F. ) ;
#12108=ORIENTED_EDGE ( 'NONE', *, *, #14922, .F. ) ;
#12113=ORIENTED_EDGE ( 'NONE', *, *, #5928, .F. ) ;
#12115=CARTESIAN_POINT ( 'NONE',  ( 172.5293059057019889, 61.25683321636181233, 7.600000000000002309 ) ) ;
#12126=EDGE_CURVE ( 'NONE', #13704, #3979, #14940, .T. ) ;
#12128=DIRECTION ( 'NONE',  ( 1.000000000000000000, 0.000000000000000000, 0.000000000000000000 ) ) ;
#12137=DIRECTION ( 'NONE',  ( -0.000000000000000000, -0.000000000000000000, 1.000000000000000000 ) ) ;
#12172=AXIS2_PLACEMENT_3D ( 'NONE', #538, #2854, #7756 ) ;
#12181=CARTESIAN_POINT ( 'NONE',  ( 15.71029453487719074, 40.04259805664093363, 10.00000000000000178 ) ) ;
#12185=VERTEX_POINT ( 'NONE', #9425 ) ;
#12197=VERTEX_POINT ( 'NONE', #3494 ) ;
#12209=ADVANCED_FACE ( 'NONE', ( #5785 ), #15479, .F. ) ;
#12215=CIRCLE ( 'NONE', #7695, 1.700000000000000178 ) ;
#12216=EDGE_LOOP ( 'NONE', ( #3281, #13684, #3330, #7792 ) ) ;
#12238=DIRECTION ( 'NONE',  ( 1.000000000000000000, 0.000000000000000000, 0.000000000000000000 ) ) ;
#12303=EDGE_LOOP ( 'NONE', ( #5024, #10813, #2890, #10229 ) ) ;
#12309=CARTESIAN_POINT ( 'NONE',  ( -34.79899788034579444, 48.72489408690345414, 10.00000000000000178 ) ) ;
#12337=AXIS2_PLACEMENT_3D ( 'NONE', #4568, #8147, #5681 ) ;
#12349=ORIENTED_EDGE ( 'NONE', *, *, #2387, .F. ) ;
#12353=ORIENTED_EDGE ( 'NONE', *, *, #1861, .F. ) ;
#12369=VECTOR ( 'NONE', #3995, 1000.000000000000000 ) ;
#12374=( NAMED_UNIT ( * ) SI_UNIT ( $, .STERADIAN. ) SOLID_ANGLE_UNIT ( ) );
#12377=DIRECTION ( 'NONE',  ( -0.000000000000000000, -0.000000000000000000, 1.000000000000000000 ) ) ;
#12403=EDGE_CURVE ( 'NONE', #8789, #457, #1511, .T. ) ;
#12431=CARTESIAN_POINT ( 'NONE',  ( -85.27455057502459113, 65.19100426474074084, 9.975000000000001421 ) ) ;
#12451=PRESENTATION_STYLE_ASSIGNMENT (( #9870 ) ) ;
#12468=FACE_OUTER_BOUND ( 'NONE', #352, .T. ) ;
#12477=CARTESIAN_POINT ( 'NONE',  ( -85.27455057502459113, 65.19100426474074084, 9.975000000000001421 ) ) ;
#12489=DIRECTION ( 'NONE',  ( -0.000000000000000000, -0.000000000000000000, 1.000000000000000000 ) ) ;
#12504=EDGE_CURVE ( 'NONE', #14396, #13094, #14506, .T. ) ;
#12505=EDGE_CURVE ( 'NONE', #935, #158, #14751, .T. ) ;
#12509=CARTESIAN_POINT ( 'NONE',  ( 172.5293059057019889, 61.25683321636181233, 10.00000000000000178 ) ) ;
#12517=EDGE_LOOP ( 'NONE', ( #4144, #5345 ) ) ;
#12528=CARTESIAN_POINT ( 'NONE',  ( 172.5293059057019889, 61.25683321636181233, 5.000000000000000000 ) ) ;
#12545=VECTOR ( 'NONE', #7087, 999.9999999999998863 ) ;
#12550=DIRECTION ( 'NONE',  ( -0.000000000000000000, -0.000000000000000000, 1.000000000000000000 ) ) ;
#12558=AXIS2_PLACEMENT_3D ( 'NONE', #3752, #5095, #1446 ) ;
#12575=ORIENTED_EDGE ( 'NONE', *, *, #9098, .T. ) ;
#12578=DIRECTION ( 'NONE',  ( -0.000000000000000000, -0.000000000000000000, 1.000000000000000000 ) ) ;
#12619=EDGE_CURVE ( 'NONE', #11858, #15074, #15229, .T. ) ;
#12643=ORIENTED_EDGE ( 'NONE', *, *, #11651, .T. ) ;
#12651=EDGE_LOOP ( 'NONE', ( #12353, #9107, #10442, #940 ) ) ;
#12677=CARTESIAN_POINT ( 'NONE',  ( 122.5806775638430253, 45.00321902537314145, 7.600000000000002309 ) ) ;
#12698=DIRECTION ( 'NONE',  ( 1.000000000000000000, 0.000000000000000000, 0.000000000000000000 ) ) ;
#12721=CARTESIAN_POINT ( 'NONE',  ( 70.26535645333922275, 38.79159067395544014, 10.00000000000000178 ) ) ;
#12722=AXIS2_PLACEMENT_3D ( 'NONE', #7144, #15321, #4675 ) ;
#12727=CARTESIAN_POINT ( 'NONE',  ( -34.79899788034579444, 48.72489408690345414, 7.600000000000002309 ) ) ;
#12746=DIRECTION ( 'NONE',  ( -0.000000000000000000, -0.000000000000000000, 1.000000000000000000 ) ) ;
#12770=CARTESIAN_POINT ( 'NONE',  ( 172.5293059057019889, 61.25683321636181233, 10.00000000000000178 ) ) ;
#12793=AXIS2_PLACEMENT_3D ( 'NONE', #9780, #354, #11201 ) ;
#12803=ORIENTED_EDGE ( 'NONE', *, *, #14066, .F. ) ;
#12813=CIRCLE ( 'NONE', #1218, 1.699999999999993072 ) ;
#12817=PRODUCT_DEFINITION_FORMATION_WITH_SPECIFIED_SOURCE ( 'ANY', '', #5635, .NOT_KNOWN. ) ;
#12823=VERTEX_POINT ( 'NONE', #10252 ) ;
#12824=DIRECTION ( 'NONE',  ( 1.000000000000000000, 0.000000000000000000, 0.000000000000000000 ) ) ;
#12831=CIRCLE ( 'NONE', #15088, 3.500000000000003109 ) ;
#12835=DIRECTION ( 'NONE',  ( -0.000000000000000000, -0.000000000000000000, 1.000000000000000000 ) ) ;
#12843=DIRECTION ( 'NONE',  ( -0.4630766004634062072, -0.8863182623094566503, 0.000000000000000000 ) ) ;
#12845=DIRECTION ( 'NONE',  ( -0.000000000000000000, 0.000000000000000000, 1.000000000000000000 ) ) ;
#12846=DIRECTION ( 'NONE',  ( 1.000000000000000000, 0.000000000000000000, 0.000000000000000000 ) ) ;
#12855=CARTESIAN_POINT ( 'NONE',  ( -31.29899788034579800, 48.72489408690345414, 9.975000000000001421 ) ) ;
#12858=AXIS2_PLACEMENT_3D ( 'NONE', #8959, #15007, #12128 ) ;
#12860=ORIENTED_EDGE ( 'NONE', *, *, #11049, .F. ) ;
#12861=VECTOR ( 'NONE', #3496, 1000.000000000000000 ) ;
#12873=ORIENTED_EDGE ( 'NONE', *, *, #4489, .T. ) ;
#12878=ORIENTED_EDGE ( 'NONE', *, *, #14885, .T. ) ;
#12887=( GEOMETRIC_REPRESENTATION_CONTEXT ( 3 ) GLOBAL_UNCERTAINTY_ASSIGNED_CONTEXT ( ( #574 ) ) GLOBAL_UNIT_ASSIGNED_CONTEXT ( ( #14890, #14737, #12374 ) ) REPRESENTATION_CONTEXT ( 'NONE', 'WORKASPACE' ) );
#12891=CARTESIAN_POINT ( 'NONE',  ( 13.88529453487718968, 40.04259805664093363, 10.00000000000000178 ) ) ;
#12900=APPLICATION_CONTEXT ( 'automotive_design' ) ;
#12901=ADVANCED_FACE ( 'NONE', ( #13792 ), #11594, .T. ) ;
#12908=DIRECTION ( 'NONE',  ( -0.000000000000000000, -0.000000000000000000, 1.000000000000000000 ) ) ;
#12913=AXIS2_PLACEMENT_3D ( 'NONE', #10816, #3778, #8604 ) ;
#12926=DIRECTION ( 'NONE',  ( 0.7071067811864983899, 0.000000000000000000, 0.7071067811865966446 ) ) ;
#12927=CARTESIAN_POINT ( 'NONE',  ( -85.27455057502459113, 65.19100426474074084, 10.00000000000000178 ) ) ;
#12930=ORIENTED_EDGE ( 'NONE', *, *, #4363, .F. ) ;
#12932=CARTESIAN_POINT ( 'NONE',  ( 119.0806775638430253, 45.00321902537314145, 9.975000000000001421 ) ) ;
#12939=VERTEX_POINT ( 'NONE', #15277 ) ;
#13015=DIRECTION ( 'NONE',  ( 1.000000000000000000, 0.000000000000000000, 0.000000000000000000 ) ) ;
#13024=AXIS2_PLACEMENT_3D ( 'NONE', #1396, #6234, #197 ) ;
#13030=CIRCLE ( 'NONE', #15048, 3.525000000000000355 ) ;
#13037=EDGE_LOOP ( 'NONE', ( #551, #8735, #12643, #14605 ) ) ;
#13047=ORIENTED_EDGE ( 'NONE', *, *, #12505, .F. ) ;
#13065=ADVANCED_FACE ( 'NONE', ( #13556 ), #1645, .F. ) ;
#13094=VERTEX_POINT ( 'NONE', #6403 ) ;
#13131=ORIENTED_EDGE ( 'NONE', *, *, #60, .T. ) ;
#13151=CARTESIAN_POINT ( 'NONE',  ( 122.5806775638430253, 45.00321902537314145, 10.00000000000000178 ) ) ;
#13159=CARTESIAN_POINT ( 'NONE',  ( -34.79899788034579444, 48.72489408690345414, 10.00000000000000178 ) ) ;
#13161=CYLINDRICAL_SURFACE ( 'NONE', #15425, 3.500000000000003109 ) ;
#13179=DIRECTION ( 'NONE',  ( 1.000000000000000000, 0.000000000000000000, 0.000000000000000000 ) ) ;
#13211=DIRECTION ( 'NONE',  ( 0.7071067811864983899, 0.000000000000000000, 0.7071067811865966446 ) ) ;
#13221=CONICAL_SURFACE ( 'NONE', #1634, 3.525000000000000355, 0.7853981633975176679 ) ;
#13244=CARTESIAN_POINT ( 'NONE',  ( 120.8806775638430224, 45.00321902537314145, 7.600000000000002309 ) ) ;
#13246=EDGE_LOOP ( 'NONE', ( #14010, #2841, #11056, #3809 ) ) ;
#13255=AXIS2_PLACEMENT_3D ( 'NONE', #7720, #6217, #2659 ) ;
#13257=DIRECTION ( 'NONE',  ( -0.000000000000000000, -0.000000000000000000, 1.000000000000000000 ) ) ;
#13263=AXIS2_PLACEMENT_3D ( 'NONE', #6760, #7952, #5332 ) ;
#13280=ORIENTED_EDGE ( 'NONE', *, *, #14143, .T. ) ;
#13293=DIRECTION ( 'NONE',  ( -0.000000000000000000, -0.000000000000000000, 1.000000000000000000 ) ) ;
#13299=CONICAL_SURFACE ( 'NONE', #12793, 3.525000000000000355, 0.7853981633973787790 ) ;
#13319=FACE_BOUND ( 'NONE', #509, .T. ) ;
#13328=CARTESIAN_POINT ( 'NONE',  ( 68.56535645333921991, 38.79159067395544014, 7.600000000000002309 ) ) ;
#13344=AXIS2_PLACEMENT_3D ( 'NONE', #8883, #6439, #1759 ) ;
#13351=CIRCLE ( 'NONE', #12858, 3.499999999999996003 ) ;
#13352=ORIENTED_EDGE ( 'NONE', *, *, #5928, .T. ) ;
#13357=EDGE_CURVE ( 'NONE', #6332, #12823, #14415, .T. ) ;
#13359=AXIS2_PLACEMENT_3D ( 'NONE', #12509, #1697, #2737 ) ;
#13362=CARTESIAN_POINT ( 'NONE',  ( 172.5293059057019889, 61.25683321636181233, 10.00000000000000178 ) ) ;
#13364=FACE_OUTER_BOUND ( 'NONE', #13037, .T. ) ;
#13373=DIRECTION ( 'NONE',  ( -0.000000000000000000, 0.000000000000000000, 1.000000000000000000 ) ) ;
#13387=DIRECTION ( 'NONE',  ( 1.000000000000000000, 0.000000000000000000, 0.000000000000000000 ) ) ;
#13390=DIRECTION ( 'NONE',  ( -0.000000000000000000, -0.000000000000000000, 1.000000000000000000 ) ) ;
#13393=CIRCLE ( 'NONE', #11135, 3.500000000000003109 ) ;
#13412=ORIENTED_EDGE ( 'NONE', *, *, #11734, .F. ) ;
#13425=VECTOR ( 'NONE', #2913, 1000.000000000000000 ) ;
#13431=CARTESIAN_POINT ( 'NONE',  ( 191.4922098844999425, 60.63967129342340456, 10.00000000000000178 ) ) ;
#13438=EDGE_LOOP ( 'NONE', ( #9316, #11471, #9974, #9091 ) ) ;
#13459=CARTESIAN_POINT ( 'NONE',  ( 169.0293059057019889, 61.25683321636181233, 10.00000000000000178 ) ) ;
#13475=DIRECTION ( 'NONE',  ( 1.000000000000000000, 0.000000000000000000, 0.000000000000000000 ) ) ;
#13520=ORIENTED_EDGE ( 'NONE', *, *, #4021, .F. ) ;
#13543=VERTEX_POINT ( 'NONE', #14649 ) ;
#13546=AXIS2_PLACEMENT_3D ( 'NONE', #14453, #5940, #3647 ) ;
#13556=FACE_OUTER_BOUND ( 'NONE', #4925, .T. ) ;
#13562=EDGE_LOOP ( 'NONE', ( #12860, #11040, #7367, #1162 ) ) ;
#13595=DIRECTION ( 'NONE',  ( 1.000000000000000000, 0.000000000000000000, 0.000000000000000000 ) ) ;
#13604=CARTESIAN_POINT ( 'NONE',  ( 20.93529453487719039, 40.04259805664093363, 10.00000000000000178 ) ) ;
#13610=CARTESIAN_POINT ( 'NONE',  ( 122.5806775638430253, 45.00321902537314145, 9.975000000000001421 ) ) ;
#13612=AXIS2_PLACEMENT_3D ( 'NONE', #9653, #2619, #14447 ) ;
#13620=CIRCLE ( 'NONE', #11363, 1.700000000000007061 ) ;
#13642=ORIENTED_EDGE ( 'NONE', *, *, #11293, .T. ) ;
#13646=EDGE_LOOP ( 'NONE', ( #11458, #7853, #1494, #13948 ) ) ;
#13656=EDGE_CURVE ( 'NONE', #7373, #3731, #13966, .T. ) ;
#13671=CARTESIAN_POINT ( 'NONE',  ( -34.79899788034579444, 48.72489408690345414, 10.00000000000000178 ) ) ;
#13684=ORIENTED_EDGE ( 'NONE', *, *, #9274, .T. ) ;
#13704=VERTEX_POINT ( 'NONE', #1873 ) ;
#13708=ORIENTED_EDGE ( 'NONE', *, *, #11049, .T. ) ;
#13716=AXIS2_PLACEMENT_3D ( 'NONE', #11764, #3315, #11689 ) ;
#13719=EDGE_CURVE ( 'NONE', #13704, #14207, #4379, .T. ) ;
#13720=AXIS2_PLACEMENT_3D ( 'NONE', #9602, #7166, #1211 ) ;
#13735=ORIENTED_EDGE ( 'NONE', *, *, #2433, .T. ) ;
#13764=DIRECTION ( 'NONE',  ( -0.000000000000000000, -0.000000000000000000, 1.000000000000000000 ) ) ;
#13772=DIRECTION ( 'NONE',  ( -0.000000000000000000, -0.000000000000000000, 1.000000000000000000 ) ) ;
#13786=VERTEX_POINT ( 'NONE', #997 ) ;
#13790=AXIS2_PLACEMENT_3D ( 'NONE', #8756, #1641, #14663 ) ;
#13792=FACE_OUTER_BOUND ( 'NONE', #14460, .T. ) ;
#13799=EDGE_CURVE ( 'NONE', #1426, #6169, #2972, .T. ) ;
#13813=ORIENTED_EDGE ( 'NONE', *, *, #14030, .T. ) ;
#13818=EDGE_CURVE ( 'NONE', #4926, #828, #1196, .T. ) ;
#13819=VECTOR ( 'NONE', #5626, 1000.000000000000000 ) ;
#13849=ADVANCED_FACE ( 'NONE', ( #2311, #5072 ), #9736, .F. ) ;
#13852=CARTESIAN_POINT ( 'NONE',  ( 174.2293059057019775, 61.25683321636181233, 7.600000000000002309 ) ) ;
#13863=ADVANCED_FACE ( 'NONE', ( #8553 ), #14530, .F. ) ;
#13869=PLANE ( 'NONE',  #6599 ) ;
#13872=VECTOR ( 'NONE', #4045, 1000.000000000000000 ) ;
#13887=CYLINDRICAL_SURFACE ( 'NONE', #2257, 1.700000000000007061 ) ;
#13891=DIRECTION ( 'NONE',  ( -0.000000000000000000, -0.000000000000000000, 1.000000000000000000 ) ) ;
#13900=ORIENTED_EDGE ( 'NONE', *, *, #4649, .F. ) ;
#13907=ORIENTED_EDGE ( 'NONE', *, *, #7733, .F. ) ;
#13914=EDGE_CURVE ( 'NONE', #9742, #6010, #6523, .T. ) ;
#13918=CARTESIAN_POINT ( 'NONE',  ( -81.74955057502458544, 65.19100426474074084, 10.00000000000000178 ) ) ;
#13946=DIRECTION ( 'NONE',  ( 0.000000000000000000, 0.000000000000000000, -1.000000000000000000 ) ) ;
#13948=ORIENTED_EDGE ( 'NONE', *, *, #14264, .T. ) ;
#13952=CARTESIAN_POINT ( 'NONE',  ( 17.41029453487719181, 40.04259805664093363, 10.00000000000000178 ) ) ;
#13965=VERTEX_POINT ( 'NONE', #7609 ) ;
#13966=CIRCLE ( 'NONE', #8930, 1.700000000000007061 ) ;
#13968=DIRECTION ( 'NONE',  ( -0.000000000000000000, -0.000000000000000000, 1.000000000000000000 ) ) ;
#13983=ORIENTED_EDGE ( 'NONE', *, *, #10730, .F. ) ;
#13986=ADVANCED_FACE ( 'NONE', ( #9976 ), #10046, .F. ) ;
#13987=AXIS2_PLACEMENT_3D ( 'NONE', #15031, #7958, #6620 ) ;
#13991=CARTESIAN_POINT ( 'NONE',  ( 169.0293059057019889, 61.25683321636181233, 7.600000000000002309 ) ) ;
#13999=VERTEX_POINT ( 'NONE', #2704 ) ;
#14010=ORIENTED_EDGE ( 'NONE', *, *, #8288, .F. ) ;
#14030=EDGE_CURVE ( 'NONE', #13094, #14396, #1698, .T. ) ;
#14049=DIRECTION ( 'NONE',  ( -0.000000000000000000, -0.000000000000000000, 1.000000000000000000 ) ) ;
#14053=ORIENTED_EDGE ( 'NONE', *, *, #1947, .T. ) ;
#14066=EDGE_CURVE ( 'NONE', #6010, #11247, #9102, .T. ) ;
#14143=EDGE_CURVE ( 'NONE', #4926, #7373, #5908, .T. ) ;
#14161=ORIENTED_EDGE ( 'NONE', *, *, #15290, .F. ) ;
#14177=DIRECTION ( 'NONE',  ( -0.000000000000000000, -0.000000000000000000, 1.000000000000000000 ) ) ;
#14180=CONICAL_SURFACE ( 'NONE', #3850, 3.525000000000000355, 0.7853981633973787790 ) ;
#14207=VERTEX_POINT ( 'NONE', #4564 ) ;
#14224=AXIS2_PLACEMENT_3D ( 'NONE', #10084, #7646, #1383 ) ;
#14248=AXIS2_PLACEMENT_3D ( 'NONE', #12477, #14049, #10438 ) ;
#14259=ADVANCED_FACE ( 'NONE', ( #10015 ), #10540, .F. ) ;
#14264=EDGE_CURVE ( 'NONE', #956, #4350, #8049, .T. ) ;
#14273=AXIS2_PLACEMENT_3D ( 'NONE', #12069, #4893, #8606 ) ;
#14287=CARTESIAN_POINT ( 'NONE',  ( 122.5806775638430253, 45.00321902537314145, 10.00000000000000178 ) ) ;
#14294=CARTESIAN_POINT ( 'NONE',  ( -111.2071507613730290, 58.10263819636593041, 10.00000000000000178 ) ) ;
#14313=LINE ( 'NONE', #7162, #15410 ) ;
#14322=VERTEX_POINT ( 'NONE', #6385 ) ;
#14323=EDGE_LOOP ( 'NONE', ( #508, #9582, #13642, #13352 ) ) ;
#14357=AXIS2_PLACEMENT_3D ( 'NONE', #1168, #3031, #4274 ) ;
#14365=ORIENTED_EDGE ( 'NONE', *, *, #2859, .T. ) ;
#14368=EDGE_LOOP ( 'NONE', ( #4203, #4183, #5964, #13983 ) ) ;
#14396=VERTEX_POINT ( 'NONE', #1783 ) ;
#14415=LINE ( 'NONE', #9535, #837 ) ;
#14416=CYLINDRICAL_SURFACE ( 'NONE', #8692, 3.500000000000003109 ) ;
#14437=LINE ( 'NONE', #1256, #273 ) ;
#14447=DIRECTION ( 'NONE',  ( 1.000000000000000000, 0.000000000000000000, 0.000000000000000000 ) ) ;
#14453=CARTESIAN_POINT ( 'NONE',  ( 181.4384305232223369, 82.69763993231136112, 10.00000000000000178 ) ) ;
#14454=EDGE_LOOP ( 'NONE', ( #3541, #2432, #14814, #2940 ) ) ;
#14460=EDGE_LOOP ( 'NONE', ( #2832, #3162, #13708, #4847 ) ) ;
#14484=VECTOR ( 'NONE', #11341, 1000.000000000000000 ) ;
#14493=CARTESIAN_POINT ( 'NONE',  ( -85.27455057502459113, 65.19100426474074084, 10.00000000000000178 ) ) ;
#14506=CIRCLE ( 'NONE', #8233, 3.499999999999999556 ) ;
#14515=ORIENTED_EDGE ( 'NONE', *, *, #1886, .T. ) ;
#14530=PLANE ( 'NONE',  #13546 ) ;
#14552=CARTESIAN_POINT ( 'NONE',  ( 122.5806775638430253, 45.00321902537314145, 10.00000000000000178 ) ) ;
#14560=EDGE_CURVE ( 'NONE', #9742, #5551, #2175, .T. ) ;
#14566=VECTOR ( 'NONE', #3173, 1000.000000000000000 ) ;
#14573=AXIS2_PLACEMENT_3D ( 'NONE', #10302, #13764, #11251 ) ;
#14600=CYLINDRICAL_SURFACE ( 'NONE', #10202, 1.700000000000007061 ) ;
#14605=ORIENTED_EDGE ( 'NONE', *, *, #4894, .F. ) ;
#14629=CONICAL_SURFACE ( 'NONE', #14880, 3.525000000000000355, 0.7853981633973787790 ) ;
#14649=CARTESIAN_POINT ( 'NONE',  ( 119.0556775638430196, 45.00321902537314145, 10.00000000000000178 ) ) ;
#14651=DIRECTION ( 'NONE',  ( -0.000000000000000000, -0.000000000000000000, -1.000000000000000000 ) ) ;
#14654=AXIS2_PLACEMENT_3D ( 'NONE', #97, #8576, #6206 ) ;
#14663=DIRECTION ( 'NONE',  ( 1.000000000000000000, 0.000000000000000000, 0.000000000000000000 ) ) ;
#14665=DIRECTION ( 'NONE',  ( 1.000000000000000000, 0.000000000000000000, 0.000000000000000000 ) ) ;
#14671=ORIENTED_EDGE ( 'NONE', *, *, #2694, .T. ) ;
#14678=EDGE_LOOP ( 'NONE', ( #4149, #10750 ) ) ;
#14684=VERTEX_POINT ( 'NONE', #7169 ) ;
#14686=DIRECTION ( 'NONE',  ( 1.000000000000000000, 0.000000000000000000, 0.000000000000000000 ) ) ;
#14719=PLANE ( 'NONE',  #11958 ) ;
#14731=CARTESIAN_POINT ( 'NONE',  ( -88.79955057502458260, 65.19100426474074084, 10.00000000000000178 ) ) ;
#14737=( NAMED_UNIT ( * ) PLANE_ANGLE_UNIT ( ) SI_UNIT ( $, .RADIAN. ) );
#14748=ORIENTED_EDGE ( 'NONE', *, *, #2039, .T. ) ;
#14751=CIRCLE ( 'NONE', #14248, 3.500000000000003109 ) ;
#14775=AXIS2_PLACEMENT_3D ( 'NONE', #9785, #8303, #4725 ) ;
#14784=CIRCLE ( 'NONE', #13790, 1.700000000000000178 ) ;
#14790=FACE_OUTER_BOUND ( 'NONE', #13246, .T. ) ;
#14798=ORIENTED_EDGE ( 'NONE', *, *, #4796, .F. ) ;
#14805=VECTOR ( 'NONE', #15070, 1000.000000000000000 ) ;
#14811=EDGE_CURVE ( 'NONE', #8410, #14322, #8059, .T. ) ;
#14814=ORIENTED_EDGE ( 'NONE', *, *, #734, .T. ) ;
#14818=ORIENTED_EDGE ( 'NONE', *, *, #8871, .T. ) ;
#14833=EDGE_LOOP ( 'NONE', ( #1862, #14161, #14515, #7730 ) ) ;
#14850=CARTESIAN_POINT ( 'NONE',  ( 126.1056775638430310, 45.00321902537314145, 10.00000000000000178 ) ) ;
#14855=CYLINDRICAL_SURFACE ( 'NONE', #2002, 3.500000000000003109 ) ;
#14858=ORIENTED_EDGE ( 'NONE', *, *, #6377, .T. ) ;
#14869=AXIS2_PLACEMENT_3D ( 'NONE', #2126, #933, #5760 ) ;
#14870=EDGE_CURVE ( 'NONE', #5551, #11247, #5264, .T. ) ;
#14880=AXIS2_PLACEMENT_3D ( 'NONE', #11222, #14911, #11376 ) ;
#14885=EDGE_CURVE ( 'NONE', #810, #7406, #15079, .T. ) ;
#14887=ORIENTED_EDGE ( 'NONE', *, *, #14066, .T. ) ;
#14889=CARTESIAN_POINT ( 'NONE',  ( -85.27455057502459113, 65.19100426474074084, 7.600000000000002309 ) ) ;
#14890=( LENGTH_UNIT ( ) NAMED_UNIT ( * ) SI_UNIT ( .MILLI., .METRE. ) );
#14895=AXIS2_PLACEMENT_3D ( 'NONE', #771, #6723, #11608 ) ;
#14901=EDGE_LOOP ( 'NONE', ( #772, #5176, #3021, #7107 ) ) ;
#14911=DIRECTION ( 'NONE',  ( -0.000000000000000000, -0.000000000000000000, 1.000000000000000000 ) ) ;
#14918=EDGE_LOOP ( 'NONE', ( #7431, #13900, #7327, #7008 ) ) ;
#14919=DIRECTION ( 'NONE',  ( -0.000000000000000000, -0.000000000000000000, 1.000000000000000000 ) ) ;
#14922=EDGE_CURVE ( 'NONE', #13965, #12005, #8556, .T. ) ;
#14924=VERTEX_POINT ( 'NONE', #7712 ) ;
#14940=LINE ( 'NONE', #15091, #9465 ) ;
#14950=DIRECTION ( 'NONE',  ( 1.000000000000000000, 0.000000000000000000, 0.000000000000000000 ) ) ;
#14962=CARTESIAN_POINT ( 'NONE',  ( 119.0556775638430196, 45.00321902537314145, 10.00000000000000178 ) ) ;
#14993=EDGE_CURVE ( 'NONE', #256, #14924, #10225, .T. ) ;
#14999=PLANE ( 'NONE',  #7051 ) ;
#15007=DIRECTION ( 'NONE',  ( -0.000000000000000000, -0.000000000000000000, 1.000000000000000000 ) ) ;
#15026=FACE_BOUND ( 'NONE', #2342, .T. ) ;
#15028=CARTESIAN_POINT ( 'NONE',  ( 17.41029453487719181, 40.04259805664093363, 10.00000000000000178 ) ) ;
#15031=CARTESIAN_POINT ( 'NONE',  ( 122.5806775638430253, 45.00321902537314145, 10.00000000000000178 ) ) ;
#15048=AXIS2_PLACEMENT_3D ( 'NONE', #13159, #10814, #51 ) ;
#15052=ORIENTED_EDGE ( 'NONE', *, *, #13357, .F. ) ;
#15053=( LENGTH_UNIT ( ) NAMED_UNIT ( * ) SI_UNIT ( .MILLI., .METRE. ) );
#15070=DIRECTION ( 'NONE',  ( -0.4147405137080060755, 0.9099397267342597129, 0.000000000000000000 ) ) ;
#15072=DIRECTION ( 'NONE',  ( 1.000000000000000000, 0.000000000000000000, 0.000000000000000000 ) ) ;
#15074=VERTEX_POINT ( 'NONE', #12891 ) ;
#15079=CIRCLE ( 'NONE', #14573, 1.700000000000007061 ) ;
#15084=DIRECTION ( 'NONE',  ( -0.000000000000000000, -0.000000000000000000, 1.000000000000000000 ) ) ;
#15088=AXIS2_PLACEMENT_3D ( 'NONE', #4758, #10929, #84 ) ;
#15091=CARTESIAN_POINT ( 'NONE',  ( 174.2293059057019775, 61.25683321636181233, 10.00000000000000178 ) ) ;
#15110=DIRECTION ( 'NONE',  ( 1.000000000000000000, 0.000000000000000000, 0.000000000000000000 ) ) ;
#15114=EDGE_LOOP ( 'NONE', ( #1620, #7210 ) ) ;
#15115=FACE_BOUND ( 'NONE', #9236, .T. ) ;
#15118=AXIS2_PLACEMENT_3D ( 'NONE', #13671, #2797, #1305 ) ;
#15154=ORIENTED_EDGE ( 'NONE', *, *, #6017, .F. ) ;
#15160=DIRECTION ( 'NONE',  ( -0.000000000000000000, -0.000000000000000000, 1.000000000000000000 ) ) ;
#15162=DIRECTION ( 'NONE',  ( 1.000000000000000000, 0.000000000000000000, 0.000000000000000000 ) ) ;
#15188=CARTESIAN_POINT ( 'NONE',  ( -34.79899788034579444, 48.72489408690345414, 10.00000000000000178 ) ) ;
#15210=CARTESIAN_POINT ( 'NONE',  ( 73.79035645333922844, 38.79159067395544014, 10.00000000000000178 ) ) ;
#15218=VERTEX_POINT ( 'NONE', #2708 ) ;
#15229=LINE ( 'NONE', #4421, #5185 ) ;
#15257=VERTEX_POINT ( 'NONE', #8557 ) ;
#15277=CARTESIAN_POINT ( 'NONE',  ( 15.71029453487719074, 40.04259805664093363, 7.600000000000002309 ) ) ;
#15290=EDGE_CURVE ( 'NONE', #8972, #12197, #12831, .T. ) ;
#15295=EDGE_LOOP ( 'NONE', ( #13131, #4705 ) ) ;
#15296=AXIS2_PLACEMENT_3D ( 'NONE', #6583, #12550, #14686 ) ;
#15321=DIRECTION ( 'NONE',  ( -0.000000000000000000, -0.000000000000000000, 1.000000000000000000 ) ) ;
#15355=ADVANCED_FACE ( 'NONE', ( #388, #6667 ), #14999, .F. ) ;
#15361=DIRECTION ( 'NONE',  ( 1.000000000000000000, 0.000000000000000000, 0.000000000000000000 ) ) ;
#15383=DIRECTION ( 'NONE',  ( -0.000000000000000000, -0.000000000000000000, 1.000000000000000000 ) ) ;
#15396=VECTOR ( 'NONE', #15445, 1000.000000000000000 ) ;
#15410=VECTOR ( 'NONE', #20, 1000.000000000000000 ) ;
#15425=AXIS2_PLACEMENT_3D ( 'NONE', #9783, #5914, #4810 ) ;
#15441=CARTESIAN_POINT ( 'NONE',  ( 17.41029453487719181, 40.04259805664093363, 10.00000000000000178 ) ) ;
#15445=DIRECTION ( 'NONE',  ( -0.4147405137080060755, 0.9099397267342597129, 0.000000000000000000 ) ) ;
#15460=ORIENTED_EDGE ( 'NONE', *, *, #14870, .T. ) ;
#15462=CIRCLE ( 'NONE', #2881, 3.500000000000003109 ) ;
#15466=ORIENTED_EDGE ( 'NONE', *, *, #13914, .T. ) ;
#15479=CYLINDRICAL_SURFACE ( 'NONE', #12722, 3.500000000000003109 ) ;
#15481=CARTESIAN_POINT ( 'NONE',  ( 68.56535645333921991, 38.79159067395544014, 5.000000000000000000 ) ) ;
#15493=ORIENTED_EDGE ( 'NONE', *, *, #218, .T. ) ;
#15498=DIRECTION ( 'NONE',  ( 0.000000000000000000, 0.000000000000000000, -1.000000000000000000 ) ) ;
#15519=DIRECTION ( 'NONE',  ( -0.000000000000000000, -0.000000000000000000, 1.000000000000000000 ) ) ;
#15540=CARTESIAN_POINT ( 'NONE',  ( -34.79899788034579444, 48.72489408690345414, 10.00000000000000178 ) ) ;
#15541=ADVANCED_FACE ( 'NONE', ( #11704 ), #11847, .F. ) ;
#15544=ORIENTED_EDGE ( 'NONE', *, *, #8964, .T. ) ;
#15548=DIRECTION ( 'NONE',  ( 0.000000000000000000, 0.000000000000000000, -1.000000000000000000 ) ) ;
#15593=DIRECTION ( 'NONE',  ( 1.000000000000000000, 0.000000000000000000, 0.000000000000000000 ) ) ;
#15607=PLANE ( 'NONE',  #14273 ) ;
#15615=VECTOR ( 'NONE', #7189, 1000.000000000000000 ) ;
#15617=ORIENTED_EDGE ( 'NONE', *, *, #8880, .T. ) ;
ENDSEC;
END-ISO-10303-21;
